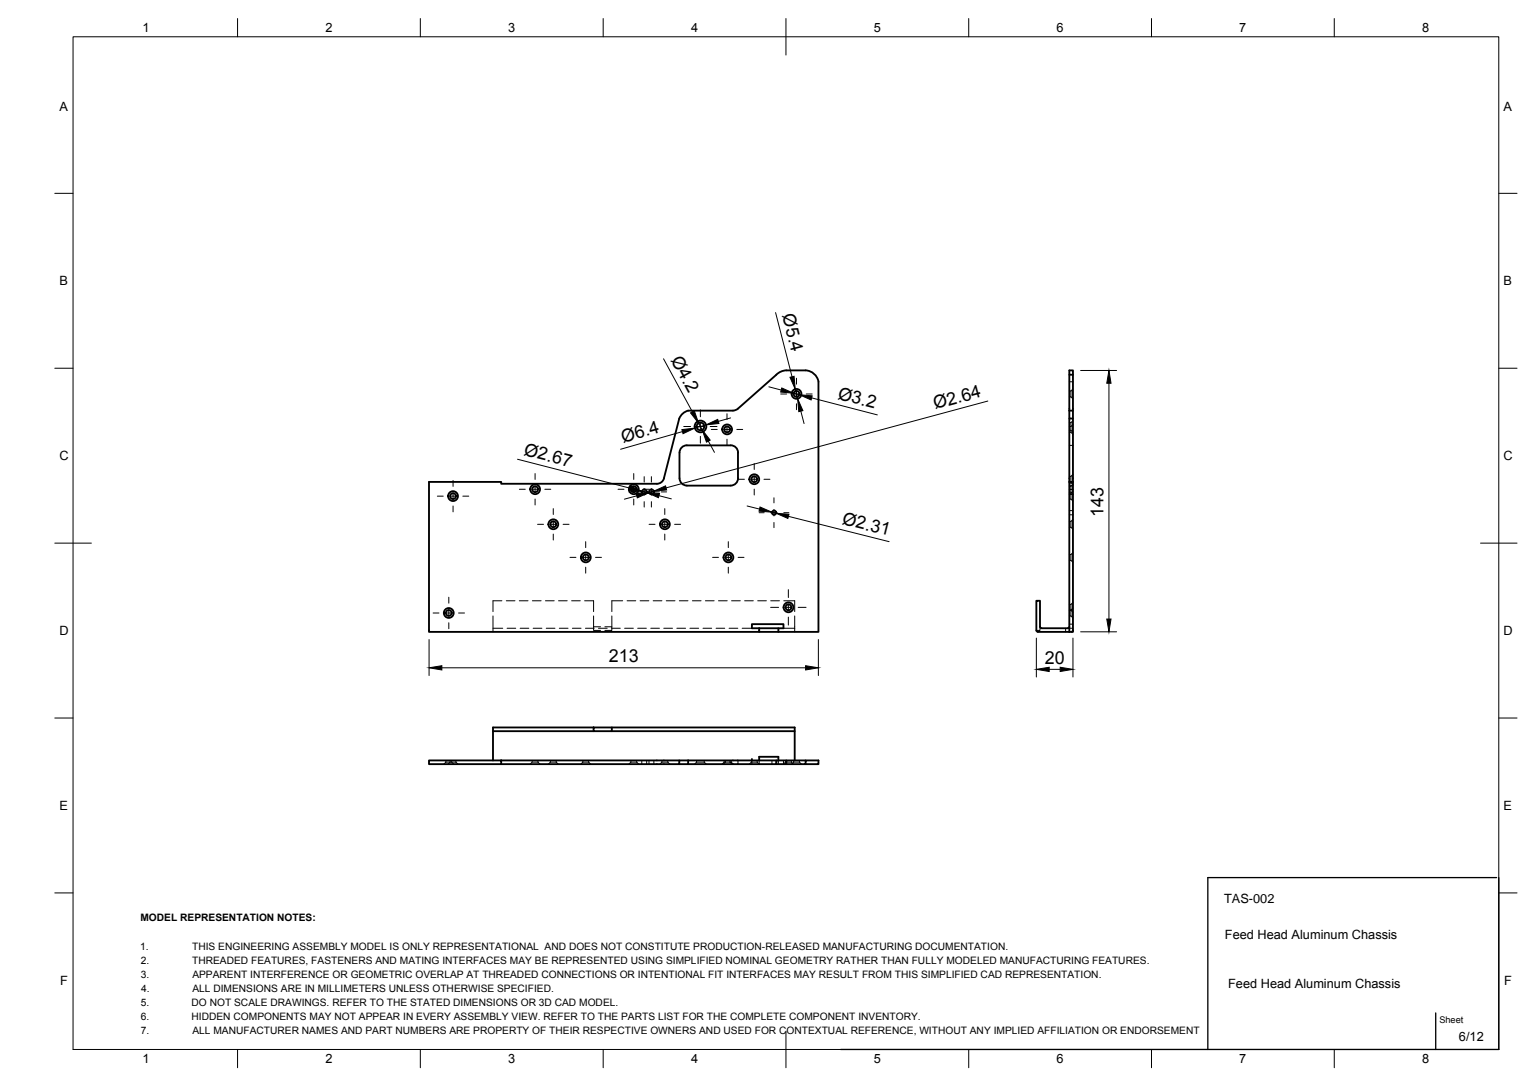
ISO-10303-21;
HEADER;
/* Generated by software containing ST-Developer
 * from STEP Tools, Inc. (www.steptools.com) 
 */

FILE_DESCRIPTION(
/* description */ ('STEP AP214'),
/* implementation_level */ '2;1');

FILE_NAME(
/* name */ 'Feed Head Aluminum Chassis.step',
/* time_stamp */ '2026-11-04T19:38:14-08:00',
/* author */ (''),
/* organization */ (''),
/* preprocessor_version */ 'ST-DEVELOPER v20.2',
/* originating_system */ 'Autodesk Translation Framework v15.17.0.0',
/* authorisation */ '');

FILE_SCHEMA (('AUTOMOTIVE_DESIGN { 1 0 10303 214 3 1 1 }'));
ENDSEC;

DATA;
#10=MECHANICAL_DESIGN_GEOMETRIC_PRESENTATION_REPRESENTATION('',(#473),#36668);
#171=CONICAL_SURFACE('',#18583,1.6,0.785398163397458);
#172=CONICAL_SURFACE('',#18587,1.6,0.785398163397457);
#173=CONICAL_SURFACE('',#18591,1.6,0.785398163397458);
#174=CONICAL_SURFACE('',#18595,1.6,0.785398163397457);
#175=CONICAL_SURFACE('',#18599,1.6,0.785398163397457);
#176=CONICAL_SURFACE('',#18603,1.6,0.785398163397457);
#177=CONICAL_SURFACE('',#18607,1.6,0.785398163397457);
#178=CONICAL_SURFACE('',#18611,1.6,0.785398163397457);
#179=CONICAL_SURFACE('',#18615,1.6,0.785398163397457);
#180=CONICAL_SURFACE('',#18619,2.1,0.785398163397457);
#181=CONICAL_SURFACE('',#18623,1.6,0.785398163397458);
#182=CONICAL_SURFACE('',#18627,1.6,0.785398163397458);
#183=CONICAL_SURFACE('',#18631,1.6,0.785398163397457);
#453=SHAPE_REPRESENTATION_RELATIONSHIP('SRR','None',#36709,#463);
#463=ADVANCED_BREP_SHAPE_REPRESENTATION('',(#483),#36661);
#473=STYLED_ITEM('',(#36768),#483);
#483=MANIFOLD_SOLID_BREP('Body1',#17796);
#585=CYLINDRICAL_SURFACE('',#18565,4.);
#586=CYLINDRICAL_SURFACE('',#18568,4.);
#587=CYLINDRICAL_SURFACE('',#18571,4.);
#588=CYLINDRICAL_SURFACE('',#18574,4.);
#589=CYLINDRICAL_SURFACE('',#18577,4.);
#590=CYLINDRICAL_SURFACE('',#18580,4.);
#591=CYLINDRICAL_SURFACE('',#18644,0.800000000000002);
#592=CYLINDRICAL_SURFACE('',#18646,0.800000000000002);
#593=CYLINDRICAL_SURFACE('',#18648,0.799999999999995);
#594=CYLINDRICAL_SURFACE('',#18651,0.799999999999995);
#595=CYLINDRICAL_SURFACE('',#18661,1.6);
#596=CYLINDRICAL_SURFACE('',#18663,1.15469920262284);
#597=CYLINDRICAL_SURFACE('',#18666,1.6);
#598=CYLINDRICAL_SURFACE('',#18668,1.6);
#599=CYLINDRICAL_SURFACE('',#18670,1.6);
#600=CYLINDRICAL_SURFACE('',#18672,1.33321558059984);
#601=CYLINDRICAL_SURFACE('',#18675,1.32106757713908);
#602=CYLINDRICAL_SURFACE('',#18678,2.1);
#603=CYLINDRICAL_SURFACE('',#18680,1.6);
#604=CYLINDRICAL_SURFACE('',#18682,1.6);
#605=CYLINDRICAL_SURFACE('',#18684,1.6);
#606=CYLINDRICAL_SURFACE('',#18686,1.6);
#607=CYLINDRICAL_SURFACE('',#18688,1.6);
#608=CYLINDRICAL_SURFACE('',#18690,1.6);
#609=CYLINDRICAL_SURFACE('',#18692,1.6);
#610=CYLINDRICAL_SURFACE('',#18694,1.6);
#611=CYLINDRICAL_SURFACE('',#18700,7.25609345692882);
#612=CYLINDRICAL_SURFACE('',#18705,8.3116573007006);
#613=CYLINDRICAL_SURFACE('',#18709,7.62932104676364);
#891=FACE_BOUND('',#2999,.T.);
#892=FACE_BOUND('',#3000,.T.);
#893=FACE_BOUND('',#3001,.T.);
#894=FACE_BOUND('',#3002,.T.);
#895=FACE_BOUND('',#3003,.T.);
#896=FACE_BOUND('',#3004,.T.);
#897=FACE_BOUND('',#3005,.T.);
#898=FACE_BOUND('',#3006,.T.);
#899=FACE_BOUND('',#3007,.T.);
#900=FACE_BOUND('',#3008,.T.);
#901=FACE_BOUND('',#3009,.T.);
#902=FACE_BOUND('',#3010,.T.);
#903=FACE_BOUND('',#3011,.T.);
#904=FACE_BOUND('',#3012,.T.);
#905=FACE_BOUND('',#3013,.T.);
#906=FACE_BOUND('',#3014,.T.);
#907=FACE_BOUND('',#3015,.T.);
#908=FACE_BOUND('',#3017,.T.);
#909=FACE_BOUND('',#3018,.T.);
#910=FACE_BOUND('',#3019,.T.);
#911=FACE_BOUND('',#3020,.T.);
#912=FACE_BOUND('',#3021,.T.);
#913=FACE_BOUND('',#3022,.T.);
#914=FACE_BOUND('',#3023,.T.);
#915=FACE_BOUND('',#3024,.T.);
#916=FACE_BOUND('',#3025,.T.);
#917=FACE_BOUND('',#3026,.T.);
#918=FACE_BOUND('',#3027,.T.);
#919=FACE_BOUND('',#3028,.T.);
#920=FACE_BOUND('',#3029,.T.);
#921=FACE_BOUND('',#3030,.T.);
#922=FACE_BOUND('',#3031,.T.);
#923=FACE_BOUND('',#3032,.T.);
#924=FACE_BOUND('',#3033,.T.);
#1255=CIRCLE('',#18566,4.);
#1256=CIRCLE('',#18567,4.);
#1257=CIRCLE('',#18569,4.);
#1258=CIRCLE('',#18570,4.);
#1259=CIRCLE('',#18572,4.);
#1260=CIRCLE('',#18573,4.);
#1261=CIRCLE('',#18575,4.);
#1262=CIRCLE('',#18576,4.);
#1263=CIRCLE('',#18578,4.);
#1264=CIRCLE('',#18579,4.);
#1265=CIRCLE('',#18581,4.);
#1266=CIRCLE('',#18582,4.);
#1267=CIRCLE('',#18584,1.6);
#1268=CIRCLE('',#18585,1.6);
#1269=CIRCLE('',#18586,2.69999999999999);
#1270=CIRCLE('',#18588,1.6);
#1271=CIRCLE('',#18589,1.6);
#1272=CIRCLE('',#18590,2.69999999999999);
#1273=CIRCLE('',#18592,1.6);
#1274=CIRCLE('',#18593,1.6);
#1275=CIRCLE('',#18594,2.7);
#1276=CIRCLE('',#18596,1.6);
#1277=CIRCLE('',#18597,1.6);
#1278=CIRCLE('',#18598,2.7);
#1279=CIRCLE('',#18600,1.6);
#1280=CIRCLE('',#18601,1.6);
#1281=CIRCLE('',#18602,2.69999999999999);
#1282=CIRCLE('',#18604,1.6);
#1283=CIRCLE('',#18605,1.6);
#1284=CIRCLE('',#18606,2.69999999999995);
#1285=CIRCLE('',#18608,1.6);
#1286=CIRCLE('',#18609,1.6);
#1287=CIRCLE('',#18610,2.7);
#1288=CIRCLE('',#18612,1.6);
#1289=CIRCLE('',#18613,1.6);
#1290=CIRCLE('',#18614,2.69999999999995);
#1291=CIRCLE('',#18616,1.6);
#1292=CIRCLE('',#18617,1.6);
#1293=CIRCLE('',#18618,2.69999999999995);
#1294=CIRCLE('',#18620,2.1);
#1295=CIRCLE('',#18621,2.1);
#1296=CIRCLE('',#18622,3.19999999999996);
#1297=CIRCLE('',#18624,1.6);
#1298=CIRCLE('',#18625,1.6);
#1299=CIRCLE('',#18626,2.7);
#1300=CIRCLE('',#18628,1.6);
#1301=CIRCLE('',#18629,1.6);
#1302=CIRCLE('',#18630,2.7);
#1303=CIRCLE('',#18632,1.6);
#1304=CIRCLE('',#18633,1.6);
#1305=CIRCLE('',#18634,2.69999999999999);
#1306=CIRCLE('',#18637,0.800000000000002);
#1307=CIRCLE('',#18638,0.800000000000002);
#1308=CIRCLE('',#18639,0.800000000000002);
#1309=CIRCLE('',#18645,0.800000000000002);
#1310=CIRCLE('',#18647,0.800000000000002);
#1311=CIRCLE('',#18649,0.800000000000002);
#1312=CIRCLE('',#18650,0.799999999999995);
#1313=CIRCLE('',#18652,0.800000000000002);
#1314=CIRCLE('',#18662,1.6);
#1315=CIRCLE('',#18664,1.15469920262284);
#1316=CIRCLE('',#18665,1.15469920262284);
#1317=CIRCLE('',#18667,1.6);
#1318=CIRCLE('',#18669,1.6);
#1319=CIRCLE('',#18671,1.6);
#1320=CIRCLE('',#18673,1.33321558059984);
#1321=CIRCLE('',#18674,1.33321558059984);
#1322=CIRCLE('',#18676,1.32106757713908);
#1323=CIRCLE('',#18677,1.32106757713908);
#1324=CIRCLE('',#18679,2.1);
#1325=CIRCLE('',#18681,1.6);
#1326=CIRCLE('',#18683,1.6);
#1327=CIRCLE('',#18685,1.6);
#1328=CIRCLE('',#18687,1.6);
#1329=CIRCLE('',#18689,1.6);
#1330=CIRCLE('',#18691,1.6);
#1331=CIRCLE('',#18693,1.6);
#1332=CIRCLE('',#18695,1.6);
#1333=CIRCLE('',#18701,7.25609345692882);
#1334=CIRCLE('',#18702,7.25609345692882);
#1335=CIRCLE('',#18706,8.3116573007006);
#1336=CIRCLE('',#18707,8.3116573007006);
#1337=CIRCLE('',#18710,7.62932104676364);
#1338=CIRCLE('',#18711,7.62932104676364);
#1880=FACE_OUTER_BOUND('',#2926,.T.);
#1881=FACE_OUTER_BOUND('',#2927,.T.);
#1882=FACE_OUTER_BOUND('',#2928,.T.);
#1883=FACE_OUTER_BOUND('',#2929,.T.);
#1884=FACE_OUTER_BOUND('',#2930,.T.);
#1885=FACE_OUTER_BOUND('',#2931,.T.);
#1886=FACE_OUTER_BOUND('',#2932,.T.);
#1887=FACE_OUTER_BOUND('',#2933,.T.);
#1888=FACE_OUTER_BOUND('',#2934,.T.);
#1889=FACE_OUTER_BOUND('',#2935,.T.);
#1890=FACE_OUTER_BOUND('',#2936,.T.);
#1891=FACE_OUTER_BOUND('',#2937,.T.);
#1892=FACE_OUTER_BOUND('',#2938,.T.);
#1893=FACE_OUTER_BOUND('',#2939,.T.);
#1894=FACE_OUTER_BOUND('',#2940,.T.);
#1895=FACE_OUTER_BOUND('',#2941,.T.);
#1896=FACE_OUTER_BOUND('',#2942,.T.);
#1897=FACE_OUTER_BOUND('',#2943,.T.);
#1898=FACE_OUTER_BOUND('',#2944,.T.);
#1899=FACE_OUTER_BOUND('',#2945,.T.);
#1900=FACE_OUTER_BOUND('',#2946,.T.);
#1901=FACE_OUTER_BOUND('',#2947,.T.);
#1902=FACE_OUTER_BOUND('',#2948,.T.);
#1903=FACE_OUTER_BOUND('',#2949,.T.);
#1904=FACE_OUTER_BOUND('',#2950,.T.);
#1905=FACE_OUTER_BOUND('',#2951,.T.);
#1906=FACE_OUTER_BOUND('',#2952,.T.);
#1907=FACE_OUTER_BOUND('',#2953,.T.);
#1908=FACE_OUTER_BOUND('',#2954,.T.);
#1909=FACE_OUTER_BOUND('',#2955,.T.);
#1910=FACE_OUTER_BOUND('',#2956,.T.);
#1911=FACE_OUTER_BOUND('',#2957,.T.);
#1912=FACE_OUTER_BOUND('',#2958,.T.);
#1913=FACE_OUTER_BOUND('',#2959,.T.);
#1914=FACE_OUTER_BOUND('',#2960,.T.);
#1915=FACE_OUTER_BOUND('',#2961,.T.);
#1916=FACE_OUTER_BOUND('',#2962,.T.);
#1917=FACE_OUTER_BOUND('',#2963,.T.);
#1918=FACE_OUTER_BOUND('',#2964,.T.);
#1919=FACE_OUTER_BOUND('',#2965,.T.);
#1920=FACE_OUTER_BOUND('',#2966,.T.);
#1921=FACE_OUTER_BOUND('',#2967,.T.);
#1922=FACE_OUTER_BOUND('',#2968,.T.);
#1923=FACE_OUTER_BOUND('',#2969,.T.);
#1924=FACE_OUTER_BOUND('',#2970,.T.);
#1925=FACE_OUTER_BOUND('',#2971,.T.);
#1926=FACE_OUTER_BOUND('',#2972,.T.);
#1927=FACE_OUTER_BOUND('',#2973,.T.);
#1928=FACE_OUTER_BOUND('',#2974,.T.);
#1929=FACE_OUTER_BOUND('',#2975,.T.);
#1930=FACE_OUTER_BOUND('',#2976,.T.);
#1931=FACE_OUTER_BOUND('',#2977,.T.);
#1932=FACE_OUTER_BOUND('',#2978,.T.);
#1933=FACE_OUTER_BOUND('',#2979,.T.);
#1934=FACE_OUTER_BOUND('',#2980,.T.);
#1935=FACE_OUTER_BOUND('',#2981,.T.);
#1936=FACE_OUTER_BOUND('',#2982,.T.);
#1937=FACE_OUTER_BOUND('',#2983,.T.);
#1938=FACE_OUTER_BOUND('',#2984,.T.);
#1939=FACE_OUTER_BOUND('',#2985,.T.);
#1940=FACE_OUTER_BOUND('',#2986,.T.);
#1941=FACE_OUTER_BOUND('',#2987,.T.);
#1942=FACE_OUTER_BOUND('',#2988,.T.);
#1943=FACE_OUTER_BOUND('',#2989,.T.);
#1944=FACE_OUTER_BOUND('',#2990,.T.);
#1945=FACE_OUTER_BOUND('',#2991,.T.);
#1946=FACE_OUTER_BOUND('',#2992,.T.);
#1947=FACE_OUTER_BOUND('',#2993,.T.);
#1948=FACE_OUTER_BOUND('',#2994,.T.);
#1949=FACE_OUTER_BOUND('',#2995,.T.);
#1950=FACE_OUTER_BOUND('',#2996,.T.);
#1951=FACE_OUTER_BOUND('',#2997,.T.);
#1952=FACE_OUTER_BOUND('',#2998,.T.);
#1953=FACE_OUTER_BOUND('',#3016,.T.);
#1954=FACE_OUTER_BOUND('',#3034,.T.);
#1955=FACE_OUTER_BOUND('',#3035,.T.);
#1956=FACE_OUTER_BOUND('',#3036,.T.);
#2926=EDGE_LOOP('',(#13188,#13189,#13190,#13191));
#2927=EDGE_LOOP('',(#13192,#13193,#13194,#13195));
#2928=EDGE_LOOP('',(#13196,#13197,#13198,#13199));
#2929=EDGE_LOOP('',(#13200,#13201,#13202,#13203));
#2930=EDGE_LOOP('',(#13204,#13205,#13206,#13207));
#2931=EDGE_LOOP('',(#13208,#13209,#13210,#13211));
#2932=EDGE_LOOP('',(#13212,#13213,#13214,#13215,#13216));
#2933=EDGE_LOOP('',(#13217,#13218,#13219,#13220,#13221));
#2934=EDGE_LOOP('',(#13222,#13223,#13224,#13225,#13226));
#2935=EDGE_LOOP('',(#13227,#13228,#13229,#13230,#13231));
#2936=EDGE_LOOP('',(#13232,#13233,#13234,#13235,#13236));
#2937=EDGE_LOOP('',(#13237,#13238,#13239,#13240,#13241));
#2938=EDGE_LOOP('',(#13242,#13243,#13244,#13245,#13246));
#2939=EDGE_LOOP('',(#13247,#13248,#13249,#13250,#13251));
#2940=EDGE_LOOP('',(#13252,#13253,#13254,#13255,#13256));
#2941=EDGE_LOOP('',(#13257,#13258,#13259,#13260,#13261));
#2942=EDGE_LOOP('',(#13262,#13263,#13264,#13265,#13266));
#2943=EDGE_LOOP('',(#13267,#13268,#13269,#13270,#13271));
#2944=EDGE_LOOP('',(#13272,#13273,#13274,#13275,#13276));
#2945=EDGE_LOOP('',(#13277,#13278,#13279,#13280));
#2946=EDGE_LOOP('',(#13281,#13282,#13283,#13284,#13285,#13286,#13287,#13288,
#13289));
#2947=EDGE_LOOP('',(#13290,#13291,#13292,#13293));
#2948=EDGE_LOOP('',(#13294,#13295,#13296,#13297,#13298));
#2949=EDGE_LOOP('',(#13299,#13300,#13301,#13302));
#2950=EDGE_LOOP('',(#13303,#13304,#13305,#13306,#13307));
#2951=EDGE_LOOP('',(#13308,#13309,#13310,#13311));
#2952=EDGE_LOOP('',(#13312,#13313,#13314,#13315,#13316,#13317));
#2953=EDGE_LOOP('',(#13318,#13319,#13320,#13321));
#2954=EDGE_LOOP('',(#13322,#13323,#13324,#13325,#13326,#13327));
#2955=EDGE_LOOP('',(#13328,#13329,#13330,#13331,#13332,#13333,#13334,#13335));
#2956=EDGE_LOOP('',(#13336,#13337,#13338,#13339));
#2957=EDGE_LOOP('',(#13340,#13341,#13342,#13343));
#2958=EDGE_LOOP('',(#13344,#13345,#13346,#13347));
#2959=EDGE_LOOP('',(#13348,#13349,#13350,#13351));
#2960=EDGE_LOOP('',(#13352,#13353,#13354,#13355));
#2961=EDGE_LOOP('',(#13356,#13357,#13358,#13359));
#2962=EDGE_LOOP('',(#13360,#13361,#13362,#13363));
#2963=EDGE_LOOP('',(#13364,#13365,#13366,#13367,#13368));
#2964=EDGE_LOOP('',(#13369,#13370,#13371,#13372));
#2965=EDGE_LOOP('',(#13373,#13374,#13375,#13376,#13377));
#2966=EDGE_LOOP('',(#13378,#13379,#13380,#13381,#13382));
#2967=EDGE_LOOP('',(#13383,#13384,#13385,#13386,#13387));
#2968=EDGE_LOOP('',(#13388,#13389,#13390,#13391));
#2969=EDGE_LOOP('',(#13392,#13393,#13394,#13395));
#2970=EDGE_LOOP('',(#13396,#13397,#13398,#13399,#13400));
#2971=EDGE_LOOP('',(#13401,#13402,#13403,#13404,#13405));
#2972=EDGE_LOOP('',(#13406,#13407,#13408,#13409,#13410));
#2973=EDGE_LOOP('',(#13411,#13412,#13413,#13414,#13415));
#2974=EDGE_LOOP('',(#13416,#13417,#13418,#13419,#13420));
#2975=EDGE_LOOP('',(#13421,#13422,#13423,#13424,#13425));
#2976=EDGE_LOOP('',(#13426,#13427,#13428,#13429,#13430));
#2977=EDGE_LOOP('',(#13431,#13432,#13433,#13434,#13435));
#2978=EDGE_LOOP('',(#13436,#13437,#13438,#13439,#13440));
#2979=EDGE_LOOP('',(#13441,#13442,#13443,#13444));
#2980=EDGE_LOOP('',(#13445,#13446,#13447,#13448));
#2981=EDGE_LOOP('',(#13449,#13450,#13451,#13452));
#2982=EDGE_LOOP('',(#13453,#13454,#13455,#13456));
#2983=EDGE_LOOP('',(#13457,#13458,#13459,#13460));
#2984=EDGE_LOOP('',(#13461,#13462,#13463,#13464));
#2985=EDGE_LOOP('',(#13465,#13466,#13467,#13468));
#2986=EDGE_LOOP('',(#13469,#13470,#13471,#13472));
#2987=EDGE_LOOP('',(#13473,#13474,#13475,#13476));
#2988=EDGE_LOOP('',(#13477,#13478,#13479,#13480));
#2989=EDGE_LOOP('',(#13481,#13482,#13483,#13484));
#2990=EDGE_LOOP('',(#13485,#13486,#13487,#13488,#13489,#13490,#13491,#13492,
#13493,#13494,#13495,#13496));
#2991=EDGE_LOOP('',(#13497,#13498,#13499,#13500));
#2992=EDGE_LOOP('',(#13501,#13502,#13503,#13504,#13505,#13506,#13507,#13508,
#13509,#13510,#13511,#13512));
#2993=EDGE_LOOP('',(#13513,#13514,#13515,#13516));
#2994=EDGE_LOOP('',(#13517,#13518,#13519,#13520));
#2995=EDGE_LOOP('',(#13521,#13522,#13523,#13524,#13525));
#2996=EDGE_LOOP('',(#13526,#13527,#13528,#13529,#13530));
#2997=EDGE_LOOP('',(#13531,#13532,#13533,#13534,#13535));
#2998=EDGE_LOOP('',(#13536,#13537,#13538,#13539,#13540,#13541,#13542,#13543,
#13544,#13545,#13546,#13547,#13548,#13549,#13550,#13551,#13552,#13553,#13554,
#13555,#13556,#13557,#13558));
#2999=EDGE_LOOP('',(#13559));
#3000=EDGE_LOOP('',(#13560,#13561,#13562,#13563,#13564,#13565,#13566,#13567));
#3001=EDGE_LOOP('',(#13568));
#3002=EDGE_LOOP('',(#13569));
#3003=EDGE_LOOP('',(#13570));
#3004=EDGE_LOOP('',(#13571));
#3005=EDGE_LOOP('',(#13572));
#3006=EDGE_LOOP('',(#13573));
#3007=EDGE_LOOP('',(#13574));
#3008=EDGE_LOOP('',(#13575));
#3009=EDGE_LOOP('',(#13576));
#3010=EDGE_LOOP('',(#13577));
#3011=EDGE_LOOP('',(#13578));
#3012=EDGE_LOOP('',(#13579));
#3013=EDGE_LOOP('',(#13580));
#3014=EDGE_LOOP('',(#13581));
#3015=EDGE_LOOP('',(#13582));
#3016=EDGE_LOOP('',(#13583,#13584,#13585,#13586,#13587,#13588,#13589,#13590,
#13591,#13592,#13593,#13594,#13595,#13596,#13597,#13598,#13599,#13600,#13601,
#13602,#13603,#13604,#13605));
#3017=EDGE_LOOP('',(#13606,#13607,#13608,#13609,#13610,#13611,#13612,#13613));
#3018=EDGE_LOOP('',(#13614));
#3019=EDGE_LOOP('',(#13615));
#3020=EDGE_LOOP('',(#13616));
#3021=EDGE_LOOP('',(#13617));
#3022=EDGE_LOOP('',(#13618));
#3023=EDGE_LOOP('',(#13619));
#3024=EDGE_LOOP('',(#13620));
#3025=EDGE_LOOP('',(#13621));
#3026=EDGE_LOOP('',(#13622));
#3027=EDGE_LOOP('',(#13623));
#3028=EDGE_LOOP('',(#13624));
#3029=EDGE_LOOP('',(#13625));
#3030=EDGE_LOOP('',(#13626));
#3031=EDGE_LOOP('',(#13627));
#3032=EDGE_LOOP('',(#13628));
#3033=EDGE_LOOP('',(#13629));
#3034=EDGE_LOOP('',(#13630,#13631,#13632,#13633));
#3035=EDGE_LOOP('',(#13634,#13635,#13636,#13637));
#3036=EDGE_LOOP('',(#13638,#13639,#13640,#13641));
#4229=LINE('',#26847,#5939);
#4230=LINE('',#26850,#5940);
#4231=LINE('',#26856,#5941);
#4232=LINE('',#26859,#5942);
#4233=LINE('',#26865,#5943);
#4234=LINE('',#26868,#5944);
#4235=LINE('',#26874,#5945);
#4236=LINE('',#26877,#5946);
#4237=LINE('',#26883,#5947);
#4238=LINE('',#26886,#5948);
#4239=LINE('',#26892,#5949);
#4240=LINE('',#26895,#5950);
#4241=LINE('',#26902,#5951);
#4242=LINE('',#26910,#5952);
#4243=LINE('',#26918,#5953);
#4244=LINE('',#26926,#5954);
#4245=LINE('',#26934,#5955);
#4246=LINE('',#26942,#5956);
#4247=LINE('',#26950,#5957);
#4248=LINE('',#26958,#5958);
#4249=LINE('',#26966,#5959);
#4250=LINE('',#26974,#5960);
#4251=LINE('',#26982,#5961);
#4252=LINE('',#26990,#5962);
#4253=LINE('',#26998,#5963);
#4254=LINE('',#27003,#5964);
#4255=LINE('',#27005,#5965);
#4256=LINE('',#27007,#5966);
#4257=LINE('',#27008,#5967);
#4258=LINE('',#27014,#5968);
#4259=LINE('',#27016,#5969);
#4260=LINE('',#27020,#5970);
#4261=LINE('',#27024,#5971);
#4262=LINE('',#27026,#5972);
#4263=LINE('',#27027,#5973);
#4264=LINE('',#27031,#5974);
#4265=LINE('',#27033,#5975);
#4266=LINE('',#27035,#5976);
#4267=LINE('',#27036,#5977);
#4268=LINE('',#27040,#5978);
#4269=LINE('',#27041,#5979);
#4270=LINE('',#27043,#5980);
#4271=LINE('',#27044,#5981);
#4272=LINE('',#27047,#5982);
#4273=LINE('',#27048,#5983);
#4274=LINE('',#27051,#5984);
#4275=LINE('',#27053,#5985);
#4276=LINE('',#27054,#5986);
#4277=LINE('',#27057,#5987);
#4278=LINE('',#27059,#5988);
#4279=LINE('',#27062,#5989);
#4280=LINE('',#27064,#5990);
#4281=LINE('',#27067,#5991);
#4282=LINE('',#27073,#5992);
#4283=LINE('',#27076,#5993);
#4284=LINE('',#27078,#5994);
#4285=LINE('',#27080,#5995);
#4286=LINE('',#27083,#5996);
#4287=LINE('',#27086,#5997);
#4288=LINE('',#27088,#5998);
#4289=LINE('',#27090,#5999);
#4290=LINE('',#27091,#6000);
#4291=LINE('',#27093,#6001);
#4292=LINE('',#27094,#6002);
#4293=LINE('',#27096,#6003);
#4294=LINE('',#27098,#6004);
#4295=LINE('',#27101,#6005);
#4296=LINE('',#27102,#6006);
#4297=LINE('',#27104,#6007);
#4298=LINE('',#27105,#6008);
#4299=LINE('',#27107,#6009);
#4300=LINE('',#27108,#6010);
#4301=LINE('',#27110,#6011);
#4302=LINE('',#27111,#6012);
#4303=LINE('',#27114,#6013);
#4304=LINE('',#27120,#6014);
#4305=LINE('',#27124,#6015);
#4306=LINE('',#27128,#6016);
#4307=LINE('',#27132,#6017);
#4308=LINE('',#27138,#6018);
#4309=LINE('',#27144,#6019);
#4310=LINE('',#27148,#6020);
#4311=LINE('',#27152,#6021);
#4312=LINE('',#27156,#6022);
#4313=LINE('',#27160,#6023);
#4314=LINE('',#27164,#6024);
#4315=LINE('',#27168,#6025);
#4316=LINE('',#27172,#6026);
#4317=LINE('',#27176,#6027);
#4318=LINE('',#27180,#6028);
#4319=LINE('',#27185,#6029);
#4320=LINE('',#27187,#6030);
#4321=LINE('',#27189,#6031);
#4322=LINE('',#27190,#6032);
#4323=LINE('',#27193,#6033);
#4324=LINE('',#27195,#6034);
#4325=LINE('',#27196,#6035);
#4326=LINE('',#27198,#6036);
#4327=LINE('',#27199,#6037);
#4328=LINE('',#27202,#6038);
#4329=LINE('',#27204,#6039);
#4330=LINE('',#27205,#6040);
#4331=LINE('',#27211,#6041);
#4332=LINE('',#27213,#6042);
#4333=LINE('',#27214,#6043);
#4334=LINE('',#27217,#6044);
#4335=LINE('',#27219,#6045);
#4336=LINE('',#27220,#6046);
#4337=LINE('',#27226,#6047);
#4338=LINE('',#27229,#6048);
#4339=LINE('',#27231,#6049);
#4340=LINE('',#27232,#6050);
#4341=LINE('',#27238,#6051);
#4342=LINE('',#27241,#6052);
#4343=LINE('',#27243,#6053);
#4344=LINE('',#27244,#6054);
#4345=LINE('',#27246,#6055);
#4346=LINE('',#27248,#6056);
#4347=LINE('',#27249,#6057);
#4348=LINE('',#27250,#6058);
#4349=LINE('',#27252,#6059);
#4350=LINE('',#27253,#6060);
#4351=LINE('',#27256,#6061);
#4352=LINE('',#27257,#6062);
#4353=LINE('',#27260,#6063);
#4354=LINE('',#27262,#6064);
#4355=LINE('',#27264,#6065);
#4356=LINE('',#27265,#6066);
#4357=LINE('',#27267,#6067);
#4358=LINE('',#27268,#6068);
#4359=LINE('',#27271,#6069);
#4360=LINE('',#27273,#6070);
#4361=LINE('',#27274,#6071);
#4362=LINE('',#27277,#6072);
#4363=LINE('',#27279,#6073);
#4364=LINE('',#27280,#6074);
#4365=LINE('',#27282,#6075);
#4366=LINE('',#27283,#6076);
#4367=LINE('',#27285,#6077);
#4368=LINE('',#27287,#6078);
#4369=LINE('',#27288,#6079);
#4370=LINE('',#27292,#6080);
#4371=LINE('',#27294,#6081);
#5939=VECTOR('',#21385,1000.);
#5940=VECTOR('',#21388,1000.);
#5941=VECTOR('',#21393,1000.);
#5942=VECTOR('',#21396,1000.);
#5943=VECTOR('',#21401,1000.);
#5944=VECTOR('',#21404,1000.);
#5945=VECTOR('',#21409,1000.);
#5946=VECTOR('',#21412,1000.);
#5947=VECTOR('',#21417,1000.);
#5948=VECTOR('',#21420,1000.);
#5949=VECTOR('',#21425,1000.);
#5950=VECTOR('',#21428,1000.);
#5951=VECTOR('',#21435,1.6);
#5952=VECTOR('',#21444,1.6);
#5953=VECTOR('',#21453,1.6);
#5954=VECTOR('',#21462,1.6);
#5955=VECTOR('',#21471,1.6);
#5956=VECTOR('',#21480,1.6);
#5957=VECTOR('',#21489,1.6);
#5958=VECTOR('',#21498,1.6);
#5959=VECTOR('',#21507,1.6);
#5960=VECTOR('',#21516,2.1);
#5961=VECTOR('',#21525,1.6);
#5962=VECTOR('',#21534,1.6);
#5963=VECTOR('',#21543,1.6);
#5964=VECTOR('',#21548,1000.);
#5965=VECTOR('',#21549,1000.);
#5966=VECTOR('',#21550,1000.);
#5967=VECTOR('',#21551,1000.);
#5968=VECTOR('',#21556,1000.);
#5969=VECTOR('',#21557,1000.);
#5970=VECTOR('',#21560,1000.);
#5971=VECTOR('',#21563,1000.);
#5972=VECTOR('',#21564,1000.);
#5973=VECTOR('',#21565,1000.);
#5974=VECTOR('',#21568,1000.);
#5975=VECTOR('',#21569,1000.);
#5976=VECTOR('',#21570,1000.);
#5977=VECTOR('',#21571,1000.);
#5978=VECTOR('',#21574,1000.);
#5979=VECTOR('',#21575,1000.);
#5980=VECTOR('',#21576,1000.);
#5981=VECTOR('',#21577,1000.);
#5982=VECTOR('',#21580,1000.);
#5983=VECTOR('',#21581,1000.);
#5984=VECTOR('',#21584,1000.);
#5985=VECTOR('',#21585,1000.);
#5986=VECTOR('',#21586,1000.);
#5987=VECTOR('',#21589,1000.);
#5988=VECTOR('',#21590,1000.);
#5989=VECTOR('',#21595,1000.);
#5990=VECTOR('',#21596,1000.);
#5991=VECTOR('',#21599,1000.);
#5992=VECTOR('',#21604,1000.);
#5993=VECTOR('',#21607,1000.);
#5994=VECTOR('',#21610,1000.);
#5995=VECTOR('',#21611,1000.);
#5996=VECTOR('',#21614,1000.);
#5997=VECTOR('',#21617,1000.);
#5998=VECTOR('',#21618,1000.);
#5999=VECTOR('',#21619,1000.);
#6000=VECTOR('',#21620,1000.);
#6001=VECTOR('',#21621,1000.);
#6002=VECTOR('',#21622,1000.);
#6003=VECTOR('',#21625,1000.);
#6004=VECTOR('',#21628,1000.);
#6005=VECTOR('',#21633,1000.);
#6006=VECTOR('',#21634,1000.);
#6007=VECTOR('',#21637,1000.);
#6008=VECTOR('',#21638,1000.);
#6009=VECTOR('',#21641,1000.);
#6010=VECTOR('',#21642,1000.);
#6011=VECTOR('',#21645,1000.);
#6012=VECTOR('',#21646,1000.);
#6013=VECTOR('',#21649,1.6);
#6014=VECTOR('',#21656,1.15469920262284);
#6015=VECTOR('',#21661,1.6);
#6016=VECTOR('',#21666,1.6);
#6017=VECTOR('',#21671,1.6);
#6018=VECTOR('',#21678,1.33321558059984);
#6019=VECTOR('',#21685,1.32106757713908);
#6020=VECTOR('',#21690,2.1);
#6021=VECTOR('',#21695,1.6);
#6022=VECTOR('',#21700,1.6);
#6023=VECTOR('',#21705,1.6);
#6024=VECTOR('',#21710,1.6);
#6025=VECTOR('',#21715,1.6);
#6026=VECTOR('',#21720,1.6);
#6027=VECTOR('',#21725,1.6);
#6028=VECTOR('',#21730,1.6);
#6029=VECTOR('',#21735,1000.);
#6030=VECTOR('',#21736,1000.);
#6031=VECTOR('',#21737,1000.);
#6032=VECTOR('',#21738,1000.);
#6033=VECTOR('',#21741,1000.);
#6034=VECTOR('',#21742,1000.);
#6035=VECTOR('',#21743,1000.);
#6036=VECTOR('',#21746,1000.);
#6037=VECTOR('',#21747,1000.);
#6038=VECTOR('',#21750,1000.);
#6039=VECTOR('',#21751,1000.);
#6040=VECTOR('',#21752,1000.);
#6041=VECTOR('',#21759,1000.);
#6042=VECTOR('',#21762,1000.);
#6043=VECTOR('',#21763,1000.);
#6044=VECTOR('',#21766,1000.);
#6045=VECTOR('',#21767,1000.);
#6046=VECTOR('',#21768,1000.);
#6047=VECTOR('',#21775,1000.);
#6048=VECTOR('',#21778,1000.);
#6049=VECTOR('',#21779,1000.);
#6050=VECTOR('',#21780,1000.);
#6051=VECTOR('',#21787,1000.);
#6052=VECTOR('',#21790,1000.);
#6053=VECTOR('',#21791,1000.);
#6054=VECTOR('',#21792,1000.);
#6055=VECTOR('',#21795,1000.);
#6056=VECTOR('',#21796,1000.);
#6057=VECTOR('',#21797,1000.);
#6058=VECTOR('',#21798,1000.);
#6059=VECTOR('',#21799,1000.);
#6060=VECTOR('',#21800,1000.);
#6061=VECTOR('',#21803,1000.);
#6062=VECTOR('',#21804,1000.);
#6063=VECTOR('',#21807,1000.);
#6064=VECTOR('',#21808,1000.);
#6065=VECTOR('',#21809,1000.);
#6066=VECTOR('',#21810,1000.);
#6067=VECTOR('',#21811,1000.);
#6068=VECTOR('',#21812,1000.);
#6069=VECTOR('',#21815,1000.);
#6070=VECTOR('',#21816,1000.);
#6071=VECTOR('',#21817,1000.);
#6072=VECTOR('',#21820,1000.);
#6073=VECTOR('',#21821,1000.);
#6074=VECTOR('',#21822,1000.);
#6075=VECTOR('',#21825,1000.);
#6076=VECTOR('',#21826,1000.);
#6077=VECTOR('',#21829,1000.);
#6078=VECTOR('',#21832,1000.);
#6079=VECTOR('',#21833,1000.);
#6080=VECTOR('',#21840,1000.);
#6081=VECTOR('',#21843,1000.);
#7633=VERTEX_POINT('',#26843);
#7634=VERTEX_POINT('',#26844);
#7635=VERTEX_POINT('',#26846);
#7636=VERTEX_POINT('',#26848);
#7637=VERTEX_POINT('',#26852);
#7638=VERTEX_POINT('',#26853);
#7639=VERTEX_POINT('',#26855);
#7640=VERTEX_POINT('',#26857);
#7641=VERTEX_POINT('',#26861);
#7642=VERTEX_POINT('',#26862);
#7643=VERTEX_POINT('',#26864);
#7644=VERTEX_POINT('',#26866);
#7645=VERTEX_POINT('',#26870);
#7646=VERTEX_POINT('',#26871);
#7647=VERTEX_POINT('',#26873);
#7648=VERTEX_POINT('',#26875);
#7649=VERTEX_POINT('',#26879);
#7650=VERTEX_POINT('',#26880);
#7651=VERTEX_POINT('',#26882);
#7652=VERTEX_POINT('',#26884);
#7653=VERTEX_POINT('',#26888);
#7654=VERTEX_POINT('',#26889);
#7655=VERTEX_POINT('',#26891);
#7656=VERTEX_POINT('',#26893);
#7657=VERTEX_POINT('',#26897);
#7658=VERTEX_POINT('',#26898);
#7659=VERTEX_POINT('',#26901);
#7660=VERTEX_POINT('',#26905);
#7661=VERTEX_POINT('',#26906);
#7662=VERTEX_POINT('',#26909);
#7663=VERTEX_POINT('',#26913);
#7664=VERTEX_POINT('',#26914);
#7665=VERTEX_POINT('',#26917);
#7666=VERTEX_POINT('',#26921);
#7667=VERTEX_POINT('',#26922);
#7668=VERTEX_POINT('',#26925);
#7669=VERTEX_POINT('',#26929);
#7670=VERTEX_POINT('',#26930);
#7671=VERTEX_POINT('',#26933);
#7672=VERTEX_POINT('',#26937);
#7673=VERTEX_POINT('',#26938);
#7674=VERTEX_POINT('',#26941);
#7675=VERTEX_POINT('',#26945);
#7676=VERTEX_POINT('',#26946);
#7677=VERTEX_POINT('',#26949);
#7678=VERTEX_POINT('',#26953);
#7679=VERTEX_POINT('',#26954);
#7680=VERTEX_POINT('',#26957);
#7681=VERTEX_POINT('',#26961);
#7682=VERTEX_POINT('',#26962);
#7683=VERTEX_POINT('',#26965);
#7684=VERTEX_POINT('',#26969);
#7685=VERTEX_POINT('',#26970);
#7686=VERTEX_POINT('',#26973);
#7687=VERTEX_POINT('',#26977);
#7688=VERTEX_POINT('',#26978);
#7689=VERTEX_POINT('',#26981);
#7690=VERTEX_POINT('',#26985);
#7691=VERTEX_POINT('',#26986);
#7692=VERTEX_POINT('',#26989);
#7693=VERTEX_POINT('',#26993);
#7694=VERTEX_POINT('',#26994);
#7695=VERTEX_POINT('',#26997);
#7696=VERTEX_POINT('',#27001);
#7697=VERTEX_POINT('',#27002);
#7698=VERTEX_POINT('',#27004);
#7699=VERTEX_POINT('',#27006);
#7700=VERTEX_POINT('',#27010);
#7701=VERTEX_POINT('',#27011);
#7702=VERTEX_POINT('',#27013);
#7703=VERTEX_POINT('',#27015);
#7704=VERTEX_POINT('',#27017);
#7705=VERTEX_POINT('',#27019);
#7706=VERTEX_POINT('',#27021);
#7707=VERTEX_POINT('',#27023);
#7708=VERTEX_POINT('',#27025);
#7709=VERTEX_POINT('',#27029);
#7710=VERTEX_POINT('',#27030);
#7711=VERTEX_POINT('',#27032);
#7712=VERTEX_POINT('',#27034);
#7713=VERTEX_POINT('',#27038);
#7714=VERTEX_POINT('',#27039);
#7715=VERTEX_POINT('',#27042);
#7716=VERTEX_POINT('',#27046);
#7717=VERTEX_POINT('',#27050);
#7718=VERTEX_POINT('',#27052);
#7719=VERTEX_POINT('',#27056);
#7720=VERTEX_POINT('',#27058);
#7721=VERTEX_POINT('',#27063);
#7722=VERTEX_POINT('',#27065);
#7723=VERTEX_POINT('',#27069);
#7724=VERTEX_POINT('',#27070);
#7725=VERTEX_POINT('',#27072);
#7726=VERTEX_POINT('',#27074);
#7727=VERTEX_POINT('',#27079);
#7728=VERTEX_POINT('',#27081);
#7729=VERTEX_POINT('',#27085);
#7730=VERTEX_POINT('',#27087);
#7731=VERTEX_POINT('',#27089);
#7732=VERTEX_POINT('',#27092);
#7733=VERTEX_POINT('',#27113);
#7734=VERTEX_POINT('',#27117);
#7735=VERTEX_POINT('',#27119);
#7736=VERTEX_POINT('',#27123);
#7737=VERTEX_POINT('',#27127);
#7738=VERTEX_POINT('',#27131);
#7739=VERTEX_POINT('',#27135);
#7740=VERTEX_POINT('',#27137);
#7741=VERTEX_POINT('',#27141);
#7742=VERTEX_POINT('',#27143);
#7743=VERTEX_POINT('',#27147);
#7744=VERTEX_POINT('',#27151);
#7745=VERTEX_POINT('',#27155);
#7746=VERTEX_POINT('',#27159);
#7747=VERTEX_POINT('',#27163);
#7748=VERTEX_POINT('',#27167);
#7749=VERTEX_POINT('',#27171);
#7750=VERTEX_POINT('',#27175);
#7751=VERTEX_POINT('',#27179);
#7752=VERTEX_POINT('',#27183);
#7753=VERTEX_POINT('',#27184);
#7754=VERTEX_POINT('',#27186);
#7755=VERTEX_POINT('',#27188);
#7756=VERTEX_POINT('',#27192);
#7757=VERTEX_POINT('',#27194);
#7758=VERTEX_POINT('',#27201);
#7759=VERTEX_POINT('',#27203);
#7760=VERTEX_POINT('',#27207);
#7761=VERTEX_POINT('',#27209);
#7762=VERTEX_POINT('',#27216);
#7763=VERTEX_POINT('',#27218);
#7764=VERTEX_POINT('',#27222);
#7765=VERTEX_POINT('',#27224);
#7766=VERTEX_POINT('',#27228);
#7767=VERTEX_POINT('',#27230);
#7768=VERTEX_POINT('',#27234);
#7769=VERTEX_POINT('',#27236);
#7770=VERTEX_POINT('',#27240);
#7771=VERTEX_POINT('',#27242);
#7772=VERTEX_POINT('',#27247);
#7773=VERTEX_POINT('',#27251);
#7774=VERTEX_POINT('',#27255);
#7775=VERTEX_POINT('',#27259);
#7776=VERTEX_POINT('',#27261);
#7777=VERTEX_POINT('',#27263);
#7778=VERTEX_POINT('',#27266);
#7779=VERTEX_POINT('',#27270);
#7780=VERTEX_POINT('',#27272);
#7781=VERTEX_POINT('',#27276);
#7782=VERTEX_POINT('',#27278);
#9646=EDGE_CURVE('',#7633,#7634,#1255,.T.);
#9647=EDGE_CURVE('',#7635,#7633,#4229,.T.);
#9648=EDGE_CURVE('',#7636,#7635,#1256,.T.);
#9649=EDGE_CURVE('',#7634,#7636,#4230,.T.);
#9650=EDGE_CURVE('',#7637,#7638,#1257,.T.);
#9651=EDGE_CURVE('',#7639,#7637,#4231,.T.);
#9652=EDGE_CURVE('',#7640,#7639,#1258,.T.);
#9653=EDGE_CURVE('',#7638,#7640,#4232,.T.);
#9654=EDGE_CURVE('',#7641,#7642,#1259,.T.);
#9655=EDGE_CURVE('',#7643,#7641,#4233,.T.);
#9656=EDGE_CURVE('',#7644,#7643,#1260,.T.);
#9657=EDGE_CURVE('',#7642,#7644,#4234,.T.);
#9658=EDGE_CURVE('',#7645,#7646,#1261,.T.);
#9659=EDGE_CURVE('',#7647,#7645,#4235,.T.);
#9660=EDGE_CURVE('',#7648,#7647,#1262,.T.);
#9661=EDGE_CURVE('',#7646,#7648,#4236,.T.);
#9662=EDGE_CURVE('',#7649,#7650,#1263,.T.);
#9663=EDGE_CURVE('',#7651,#7649,#4237,.T.);
#9664=EDGE_CURVE('',#7652,#7651,#1264,.T.);
#9665=EDGE_CURVE('',#7650,#7652,#4238,.T.);
#9666=EDGE_CURVE('',#7653,#7654,#1265,.T.);
#9667=EDGE_CURVE('',#7655,#7653,#4239,.T.);
#9668=EDGE_CURVE('',#7656,#7655,#1266,.T.);
#9669=EDGE_CURVE('',#7654,#7656,#4240,.T.);
#9670=EDGE_CURVE('',#7657,#7658,#1267,.T.);
#9671=EDGE_CURVE('',#7658,#7657,#1268,.T.);
#9672=EDGE_CURVE('',#7658,#7659,#4241,.T.);
#9673=EDGE_CURVE('',#7659,#7659,#1269,.T.);
#9674=EDGE_CURVE('',#7660,#7661,#1270,.T.);
#9675=EDGE_CURVE('',#7661,#7660,#1271,.T.);
#9676=EDGE_CURVE('',#7661,#7662,#4242,.T.);
#9677=EDGE_CURVE('',#7662,#7662,#1272,.T.);
#9678=EDGE_CURVE('',#7663,#7664,#1273,.T.);
#9679=EDGE_CURVE('',#7664,#7663,#1274,.T.);
#9680=EDGE_CURVE('',#7664,#7665,#4243,.T.);
#9681=EDGE_CURVE('',#7665,#7665,#1275,.T.);
#9682=EDGE_CURVE('',#7666,#7667,#1276,.T.);
#9683=EDGE_CURVE('',#7667,#7666,#1277,.T.);
#9684=EDGE_CURVE('',#7667,#7668,#4244,.T.);
#9685=EDGE_CURVE('',#7668,#7668,#1278,.T.);
#9686=EDGE_CURVE('',#7669,#7670,#1279,.T.);
#9687=EDGE_CURVE('',#7670,#7669,#1280,.T.);
#9688=EDGE_CURVE('',#7670,#7671,#4245,.T.);
#9689=EDGE_CURVE('',#7671,#7671,#1281,.T.);
#9690=EDGE_CURVE('',#7672,#7673,#1282,.T.);
#9691=EDGE_CURVE('',#7673,#7672,#1283,.T.);
#9692=EDGE_CURVE('',#7673,#7674,#4246,.T.);
#9693=EDGE_CURVE('',#7674,#7674,#1284,.T.);
#9694=EDGE_CURVE('',#7675,#7676,#1285,.T.);
#9695=EDGE_CURVE('',#7676,#7675,#1286,.T.);
#9696=EDGE_CURVE('',#7676,#7677,#4247,.T.);
#9697=EDGE_CURVE('',#7677,#7677,#1287,.T.);
#9698=EDGE_CURVE('',#7678,#7679,#1288,.T.);
#9699=EDGE_CURVE('',#7679,#7678,#1289,.T.);
#9700=EDGE_CURVE('',#7679,#7680,#4248,.T.);
#9701=EDGE_CURVE('',#7680,#7680,#1290,.T.);
#9702=EDGE_CURVE('',#7681,#7682,#1291,.T.);
#9703=EDGE_CURVE('',#7682,#7681,#1292,.T.);
#9704=EDGE_CURVE('',#7682,#7683,#4249,.T.);
#9705=EDGE_CURVE('',#7683,#7683,#1293,.T.);
#9706=EDGE_CURVE('',#7684,#7685,#1294,.T.);
#9707=EDGE_CURVE('',#7685,#7684,#1295,.T.);
#9708=EDGE_CURVE('',#7685,#7686,#4250,.T.);
#9709=EDGE_CURVE('',#7686,#7686,#1296,.T.);
#9710=EDGE_CURVE('',#7687,#7688,#1297,.T.);
#9711=EDGE_CURVE('',#7688,#7687,#1298,.T.);
#9712=EDGE_CURVE('',#7688,#7689,#4251,.T.);
#9713=EDGE_CURVE('',#7689,#7689,#1299,.T.);
#9714=EDGE_CURVE('',#7690,#7691,#1300,.T.);
#9715=EDGE_CURVE('',#7691,#7690,#1301,.T.);
#9716=EDGE_CURVE('',#7691,#7692,#4252,.T.);
#9717=EDGE_CURVE('',#7692,#7692,#1302,.T.);
#9718=EDGE_CURVE('',#7693,#7694,#1303,.T.);
#9719=EDGE_CURVE('',#7694,#7693,#1304,.T.);
#9720=EDGE_CURVE('',#7694,#7695,#4253,.T.);
#9721=EDGE_CURVE('',#7695,#7695,#1305,.T.);
#9722=EDGE_CURVE('',#7696,#7697,#4254,.T.);
#9723=EDGE_CURVE('',#7697,#7698,#4255,.T.);
#9724=EDGE_CURVE('',#7698,#7699,#4256,.T.);
#9725=EDGE_CURVE('',#7699,#7696,#4257,.T.);
#9726=EDGE_CURVE('',#7700,#7701,#1306,.T.);
#9727=EDGE_CURVE('',#7702,#7701,#4258,.T.);
#9728=EDGE_CURVE('',#7703,#7702,#4259,.T.);
#9729=EDGE_CURVE('',#7704,#7703,#1307,.T.);
#9730=EDGE_CURVE('',#7705,#7704,#4260,.T.);
#9731=EDGE_CURVE('',#7706,#7705,#1308,.T.);
#9732=EDGE_CURVE('',#7706,#7707,#4261,.T.);
#9733=EDGE_CURVE('',#7707,#7708,#4262,.T.);
#9734=EDGE_CURVE('',#7708,#7700,#4263,.T.);
#9735=EDGE_CURVE('',#7709,#7710,#4264,.T.);
#9736=EDGE_CURVE('',#7710,#7711,#4265,.T.);
#9737=EDGE_CURVE('',#7711,#7712,#4266,.T.);
#9738=EDGE_CURVE('',#7712,#7709,#4267,.T.);
#9739=EDGE_CURVE('',#7713,#7714,#4268,.T.);
#9740=EDGE_CURVE('',#7711,#7714,#4269,.T.);
#9741=EDGE_CURVE('',#7715,#7710,#4270,.T.);
#9742=EDGE_CURVE('',#7715,#7713,#4271,.T.);
#9743=EDGE_CURVE('',#7714,#7716,#4272,.T.);
#9744=EDGE_CURVE('',#7712,#7716,#4273,.T.);
#9745=EDGE_CURVE('',#7716,#7717,#4274,.T.);
#9746=EDGE_CURVE('',#7718,#7717,#4275,.T.);
#9747=EDGE_CURVE('',#7709,#7718,#4276,.T.);
#9748=EDGE_CURVE('',#7704,#7719,#4277,.T.);
#9749=EDGE_CURVE('',#7720,#7703,#4278,.T.);
#9750=EDGE_CURVE('',#7719,#7720,#1309,.T.);
#9751=EDGE_CURVE('',#7706,#7709,#4279,.T.);
#9752=EDGE_CURVE('',#7721,#7705,#4280,.T.);
#9753=EDGE_CURVE('',#7722,#7721,#1310,.T.);
#9754=EDGE_CURVE('',#7710,#7722,#4281,.T.);
#9755=EDGE_CURVE('',#7723,#7724,#1311,.T.);
#9756=EDGE_CURVE('',#7725,#7723,#4282,.T.);
#9757=EDGE_CURVE('',#7726,#7725,#1312,.T.);
#9758=EDGE_CURVE('',#7724,#7726,#4283,.T.);
#9759=EDGE_CURVE('',#7716,#7700,#4284,.T.);
#9760=EDGE_CURVE('',#7727,#7714,#4285,.T.);
#9761=EDGE_CURVE('',#7728,#7727,#1313,.T.);
#9762=EDGE_CURVE('',#7701,#7728,#4286,.T.);
#9763=EDGE_CURVE('',#7728,#7729,#4287,.T.);
#9764=EDGE_CURVE('',#7730,#7727,#4288,.T.);
#9765=EDGE_CURVE('',#7731,#7730,#4289,.T.);
#9766=EDGE_CURVE('',#7722,#7731,#4290,.T.);
#9767=EDGE_CURVE('',#7732,#7721,#4291,.T.);
#9768=EDGE_CURVE('',#7729,#7732,#4292,.T.);
#9769=EDGE_CURVE('',#7731,#7715,#4293,.T.);
#9770=EDGE_CURVE('',#7730,#7713,#4294,.T.);
#9771=EDGE_CURVE('',#7647,#7636,#4295,.T.);
#9772=EDGE_CURVE('',#7645,#7634,#4296,.T.);
#9773=EDGE_CURVE('',#7641,#7646,#4297,.T.);
#9774=EDGE_CURVE('',#7643,#7648,#4298,.T.);
#9775=EDGE_CURVE('',#7637,#7642,#4299,.T.);
#9776=EDGE_CURVE('',#7639,#7644,#4300,.T.);
#9777=EDGE_CURVE('',#7633,#7638,#4301,.T.);
#9778=EDGE_CURVE('',#7635,#7640,#4302,.T.);
#9779=EDGE_CURVE('',#7693,#7733,#4303,.T.);
#9780=EDGE_CURVE('',#7733,#7733,#1314,.T.);
#9781=EDGE_CURVE('',#7734,#7734,#1315,.T.);
#9782=EDGE_CURVE('',#7734,#7735,#4304,.T.);
#9783=EDGE_CURVE('',#7735,#7735,#1316,.T.);
#9784=EDGE_CURVE('',#7687,#7736,#4305,.T.);
#9785=EDGE_CURVE('',#7736,#7736,#1317,.T.);
#9786=EDGE_CURVE('',#7675,#7737,#4306,.T.);
#9787=EDGE_CURVE('',#7737,#7737,#1318,.T.);
#9788=EDGE_CURVE('',#7690,#7738,#4307,.T.);
#9789=EDGE_CURVE('',#7738,#7738,#1319,.T.);
#9790=EDGE_CURVE('',#7739,#7739,#1320,.T.);
#9791=EDGE_CURVE('',#7739,#7740,#4308,.T.);
#9792=EDGE_CURVE('',#7740,#7740,#1321,.T.);
#9793=EDGE_CURVE('',#7741,#7741,#1322,.T.);
#9794=EDGE_CURVE('',#7741,#7742,#4309,.T.);
#9795=EDGE_CURVE('',#7742,#7742,#1323,.T.);
#9796=EDGE_CURVE('',#7684,#7743,#4310,.T.);
#9797=EDGE_CURVE('',#7743,#7743,#1324,.T.);
#9798=EDGE_CURVE('',#7672,#7744,#4311,.T.);
#9799=EDGE_CURVE('',#7744,#7744,#1325,.T.);
#9800=EDGE_CURVE('',#7681,#7745,#4312,.T.);
#9801=EDGE_CURVE('',#7745,#7745,#1326,.T.);
#9802=EDGE_CURVE('',#7678,#7746,#4313,.T.);
#9803=EDGE_CURVE('',#7746,#7746,#1327,.T.);
#9804=EDGE_CURVE('',#7669,#7747,#4314,.T.);
#9805=EDGE_CURVE('',#7747,#7747,#1328,.T.);
#9806=EDGE_CURVE('',#7666,#7748,#4315,.T.);
#9807=EDGE_CURVE('',#7748,#7748,#1329,.T.);
#9808=EDGE_CURVE('',#7663,#7749,#4316,.T.);
#9809=EDGE_CURVE('',#7749,#7749,#1330,.T.);
#9810=EDGE_CURVE('',#7657,#7750,#4317,.T.);
#9811=EDGE_CURVE('',#7750,#7750,#1331,.T.);
#9812=EDGE_CURVE('',#7660,#7751,#4318,.T.);
#9813=EDGE_CURVE('',#7751,#7751,#1332,.T.);
#9814=EDGE_CURVE('',#7752,#7753,#4319,.T.);
#9815=EDGE_CURVE('',#7754,#7753,#4320,.T.);
#9816=EDGE_CURVE('',#7755,#7754,#4321,.T.);
#9817=EDGE_CURVE('',#7755,#7752,#4322,.T.);
#9818=EDGE_CURVE('',#7756,#7752,#4323,.T.);
#9819=EDGE_CURVE('',#7757,#7755,#4324,.T.);
#9820=EDGE_CURVE('',#7757,#7756,#4325,.T.);
#9821=EDGE_CURVE('',#7650,#7757,#4326,.T.);
#9822=EDGE_CURVE('',#7652,#7756,#4327,.T.);
#9823=EDGE_CURVE('',#7758,#7651,#4328,.T.);
#9824=EDGE_CURVE('',#7759,#7649,#4329,.T.);
#9825=EDGE_CURVE('',#7759,#7758,#4330,.T.);
#9826=EDGE_CURVE('',#7760,#7758,#1333,.T.);
#9827=EDGE_CURVE('',#7761,#7759,#1334,.T.);
#9828=EDGE_CURVE('',#7761,#7760,#4331,.T.);
#9829=EDGE_CURVE('',#7654,#7761,#4332,.T.);
#9830=EDGE_CURVE('',#7656,#7760,#4333,.T.);
#9831=EDGE_CURVE('',#7762,#7655,#4334,.T.);
#9832=EDGE_CURVE('',#7763,#7653,#4335,.T.);
#9833=EDGE_CURVE('',#7763,#7762,#4336,.T.);
#9834=EDGE_CURVE('',#7764,#7762,#1335,.T.);
#9835=EDGE_CURVE('',#7765,#7763,#1336,.T.);
#9836=EDGE_CURVE('',#7765,#7764,#4337,.T.);
#9837=EDGE_CURVE('',#7766,#7764,#4338,.T.);
#9838=EDGE_CURVE('',#7767,#7765,#4339,.T.);
#9839=EDGE_CURVE('',#7767,#7766,#4340,.T.);
#9840=EDGE_CURVE('',#7768,#7766,#1337,.T.);
#9841=EDGE_CURVE('',#7769,#7767,#1338,.T.);
#9842=EDGE_CURVE('',#7769,#7768,#4341,.T.);
#9843=EDGE_CURVE('',#7770,#7768,#4342,.T.);
#9844=EDGE_CURVE('',#7771,#7769,#4343,.T.);
#9845=EDGE_CURVE('',#7771,#7770,#4344,.T.);
#9846=EDGE_CURVE('',#7725,#7697,#4345,.T.);
#9847=EDGE_CURVE('',#7723,#7772,#4346,.T.);
#9848=EDGE_CURVE('',#7702,#7772,#4347,.T.);
#9849=EDGE_CURVE('',#7729,#7770,#4348,.T.);
#9850=EDGE_CURVE('',#7773,#7771,#4349,.T.);
#9851=EDGE_CURVE('',#7773,#7698,#4350,.T.);
#9852=EDGE_CURVE('',#7774,#7699,#4351,.T.);
#9853=EDGE_CURVE('',#7774,#7773,#4352,.T.);
#9854=EDGE_CURVE('',#7775,#7696,#4353,.T.);
#9855=EDGE_CURVE('',#7776,#7774,#4354,.T.);
#9856=EDGE_CURVE('',#7776,#7777,#4355,.T.);
#9857=EDGE_CURVE('',#7732,#7777,#4356,.T.);
#9858=EDGE_CURVE('',#7778,#7719,#4357,.T.);
#9859=EDGE_CURVE('',#7775,#7778,#4358,.T.);
#9860=EDGE_CURVE('',#7779,#7777,#4359,.T.);
#9861=EDGE_CURVE('',#7780,#7776,#4360,.T.);
#9862=EDGE_CURVE('',#7780,#7779,#4361,.T.);
#9863=EDGE_CURVE('',#7781,#7779,#4362,.T.);
#9864=EDGE_CURVE('',#7782,#7780,#4363,.T.);
#9865=EDGE_CURVE('',#7782,#7781,#4364,.T.);
#9866=EDGE_CURVE('',#7720,#7781,#4365,.T.);
#9867=EDGE_CURVE('',#7778,#7782,#4366,.T.);
#9868=EDGE_CURVE('',#7726,#7775,#4367,.T.);
#9869=EDGE_CURVE('',#7753,#7772,#4368,.T.);
#9870=EDGE_CURVE('',#7754,#7724,#4369,.T.);
#9871=EDGE_CURVE('',#7718,#7707,#4370,.T.);
#9872=EDGE_CURVE('',#7717,#7708,#4371,.T.);
#13188=ORIENTED_EDGE('',*,*,#9646,.F.);
#13189=ORIENTED_EDGE('',*,*,#9647,.F.);
#13190=ORIENTED_EDGE('',*,*,#9648,.F.);
#13191=ORIENTED_EDGE('',*,*,#9649,.F.);
#13192=ORIENTED_EDGE('',*,*,#9650,.F.);
#13193=ORIENTED_EDGE('',*,*,#9651,.F.);
#13194=ORIENTED_EDGE('',*,*,#9652,.F.);
#13195=ORIENTED_EDGE('',*,*,#9653,.F.);
#13196=ORIENTED_EDGE('',*,*,#9654,.F.);
#13197=ORIENTED_EDGE('',*,*,#9655,.F.);
#13198=ORIENTED_EDGE('',*,*,#9656,.F.);
#13199=ORIENTED_EDGE('',*,*,#9657,.F.);
#13200=ORIENTED_EDGE('',*,*,#9658,.F.);
#13201=ORIENTED_EDGE('',*,*,#9659,.F.);
#13202=ORIENTED_EDGE('',*,*,#9660,.F.);
#13203=ORIENTED_EDGE('',*,*,#9661,.F.);
#13204=ORIENTED_EDGE('',*,*,#9662,.F.);
#13205=ORIENTED_EDGE('',*,*,#9663,.F.);
#13206=ORIENTED_EDGE('',*,*,#9664,.F.);
#13207=ORIENTED_EDGE('',*,*,#9665,.F.);
#13208=ORIENTED_EDGE('',*,*,#9666,.F.);
#13209=ORIENTED_EDGE('',*,*,#9667,.F.);
#13210=ORIENTED_EDGE('',*,*,#9668,.F.);
#13211=ORIENTED_EDGE('',*,*,#9669,.F.);
#13212=ORIENTED_EDGE('',*,*,#9670,.F.);
#13213=ORIENTED_EDGE('',*,*,#9671,.F.);
#13214=ORIENTED_EDGE('',*,*,#9672,.T.);
#13215=ORIENTED_EDGE('',*,*,#9673,.F.);
#13216=ORIENTED_EDGE('',*,*,#9672,.F.);
#13217=ORIENTED_EDGE('',*,*,#9674,.F.);
#13218=ORIENTED_EDGE('',*,*,#9675,.F.);
#13219=ORIENTED_EDGE('',*,*,#9676,.T.);
#13220=ORIENTED_EDGE('',*,*,#9677,.F.);
#13221=ORIENTED_EDGE('',*,*,#9676,.F.);
#13222=ORIENTED_EDGE('',*,*,#9678,.F.);
#13223=ORIENTED_EDGE('',*,*,#9679,.F.);
#13224=ORIENTED_EDGE('',*,*,#9680,.T.);
#13225=ORIENTED_EDGE('',*,*,#9681,.F.);
#13226=ORIENTED_EDGE('',*,*,#9680,.F.);
#13227=ORIENTED_EDGE('',*,*,#9682,.F.);
#13228=ORIENTED_EDGE('',*,*,#9683,.F.);
#13229=ORIENTED_EDGE('',*,*,#9684,.T.);
#13230=ORIENTED_EDGE('',*,*,#9685,.F.);
#13231=ORIENTED_EDGE('',*,*,#9684,.F.);
#13232=ORIENTED_EDGE('',*,*,#9686,.F.);
#13233=ORIENTED_EDGE('',*,*,#9687,.F.);
#13234=ORIENTED_EDGE('',*,*,#9688,.T.);
#13235=ORIENTED_EDGE('',*,*,#9689,.F.);
#13236=ORIENTED_EDGE('',*,*,#9688,.F.);
#13237=ORIENTED_EDGE('',*,*,#9690,.F.);
#13238=ORIENTED_EDGE('',*,*,#9691,.F.);
#13239=ORIENTED_EDGE('',*,*,#9692,.T.);
#13240=ORIENTED_EDGE('',*,*,#9693,.F.);
#13241=ORIENTED_EDGE('',*,*,#9692,.F.);
#13242=ORIENTED_EDGE('',*,*,#9694,.F.);
#13243=ORIENTED_EDGE('',*,*,#9695,.F.);
#13244=ORIENTED_EDGE('',*,*,#9696,.T.);
#13245=ORIENTED_EDGE('',*,*,#9697,.F.);
#13246=ORIENTED_EDGE('',*,*,#9696,.F.);
#13247=ORIENTED_EDGE('',*,*,#9698,.F.);
#13248=ORIENTED_EDGE('',*,*,#9699,.F.);
#13249=ORIENTED_EDGE('',*,*,#9700,.T.);
#13250=ORIENTED_EDGE('',*,*,#9701,.F.);
#13251=ORIENTED_EDGE('',*,*,#9700,.F.);
#13252=ORIENTED_EDGE('',*,*,#9702,.F.);
#13253=ORIENTED_EDGE('',*,*,#9703,.F.);
#13254=ORIENTED_EDGE('',*,*,#9704,.T.);
#13255=ORIENTED_EDGE('',*,*,#9705,.F.);
#13256=ORIENTED_EDGE('',*,*,#9704,.F.);
#13257=ORIENTED_EDGE('',*,*,#9706,.F.);
#13258=ORIENTED_EDGE('',*,*,#9707,.F.);
#13259=ORIENTED_EDGE('',*,*,#9708,.T.);
#13260=ORIENTED_EDGE('',*,*,#9709,.F.);
#13261=ORIENTED_EDGE('',*,*,#9708,.F.);
#13262=ORIENTED_EDGE('',*,*,#9710,.F.);
#13263=ORIENTED_EDGE('',*,*,#9711,.F.);
#13264=ORIENTED_EDGE('',*,*,#9712,.T.);
#13265=ORIENTED_EDGE('',*,*,#9713,.F.);
#13266=ORIENTED_EDGE('',*,*,#9712,.F.);
#13267=ORIENTED_EDGE('',*,*,#9714,.F.);
#13268=ORIENTED_EDGE('',*,*,#9715,.F.);
#13269=ORIENTED_EDGE('',*,*,#9716,.T.);
#13270=ORIENTED_EDGE('',*,*,#9717,.F.);
#13271=ORIENTED_EDGE('',*,*,#9716,.F.);
#13272=ORIENTED_EDGE('',*,*,#9718,.F.);
#13273=ORIENTED_EDGE('',*,*,#9719,.F.);
#13274=ORIENTED_EDGE('',*,*,#9720,.T.);
#13275=ORIENTED_EDGE('',*,*,#9721,.F.);
#13276=ORIENTED_EDGE('',*,*,#9720,.F.);
#13277=ORIENTED_EDGE('',*,*,#9722,.T.);
#13278=ORIENTED_EDGE('',*,*,#9723,.T.);
#13279=ORIENTED_EDGE('',*,*,#9724,.T.);
#13280=ORIENTED_EDGE('',*,*,#9725,.T.);
#13281=ORIENTED_EDGE('',*,*,#9726,.T.);
#13282=ORIENTED_EDGE('',*,*,#9727,.F.);
#13283=ORIENTED_EDGE('',*,*,#9728,.F.);
#13284=ORIENTED_EDGE('',*,*,#9729,.F.);
#13285=ORIENTED_EDGE('',*,*,#9730,.F.);
#13286=ORIENTED_EDGE('',*,*,#9731,.F.);
#13287=ORIENTED_EDGE('',*,*,#9732,.T.);
#13288=ORIENTED_EDGE('',*,*,#9733,.T.);
#13289=ORIENTED_EDGE('',*,*,#9734,.T.);
#13290=ORIENTED_EDGE('',*,*,#9735,.T.);
#13291=ORIENTED_EDGE('',*,*,#9736,.T.);
#13292=ORIENTED_EDGE('',*,*,#9737,.T.);
#13293=ORIENTED_EDGE('',*,*,#9738,.T.);
#13294=ORIENTED_EDGE('',*,*,#9739,.T.);
#13295=ORIENTED_EDGE('',*,*,#9740,.F.);
#13296=ORIENTED_EDGE('',*,*,#9736,.F.);
#13297=ORIENTED_EDGE('',*,*,#9741,.F.);
#13298=ORIENTED_EDGE('',*,*,#9742,.T.);
#13299=ORIENTED_EDGE('',*,*,#9743,.T.);
#13300=ORIENTED_EDGE('',*,*,#9744,.F.);
#13301=ORIENTED_EDGE('',*,*,#9737,.F.);
#13302=ORIENTED_EDGE('',*,*,#9740,.T.);
#13303=ORIENTED_EDGE('',*,*,#9745,.T.);
#13304=ORIENTED_EDGE('',*,*,#9746,.F.);
#13305=ORIENTED_EDGE('',*,*,#9747,.F.);
#13306=ORIENTED_EDGE('',*,*,#9738,.F.);
#13307=ORIENTED_EDGE('',*,*,#9744,.T.);
#13308=ORIENTED_EDGE('',*,*,#9748,.F.);
#13309=ORIENTED_EDGE('',*,*,#9729,.T.);
#13310=ORIENTED_EDGE('',*,*,#9749,.F.);
#13311=ORIENTED_EDGE('',*,*,#9750,.F.);
#13312=ORIENTED_EDGE('',*,*,#9751,.F.);
#13313=ORIENTED_EDGE('',*,*,#9731,.T.);
#13314=ORIENTED_EDGE('',*,*,#9752,.F.);
#13315=ORIENTED_EDGE('',*,*,#9753,.F.);
#13316=ORIENTED_EDGE('',*,*,#9754,.F.);
#13317=ORIENTED_EDGE('',*,*,#9735,.F.);
#13318=ORIENTED_EDGE('',*,*,#9755,.F.);
#13319=ORIENTED_EDGE('',*,*,#9756,.F.);
#13320=ORIENTED_EDGE('',*,*,#9757,.F.);
#13321=ORIENTED_EDGE('',*,*,#9758,.F.);
#13322=ORIENTED_EDGE('',*,*,#9726,.F.);
#13323=ORIENTED_EDGE('',*,*,#9759,.F.);
#13324=ORIENTED_EDGE('',*,*,#9743,.F.);
#13325=ORIENTED_EDGE('',*,*,#9760,.F.);
#13326=ORIENTED_EDGE('',*,*,#9761,.F.);
#13327=ORIENTED_EDGE('',*,*,#9762,.F.);
#13328=ORIENTED_EDGE('',*,*,#9763,.F.);
#13329=ORIENTED_EDGE('',*,*,#9761,.T.);
#13330=ORIENTED_EDGE('',*,*,#9764,.F.);
#13331=ORIENTED_EDGE('',*,*,#9765,.F.);
#13332=ORIENTED_EDGE('',*,*,#9766,.F.);
#13333=ORIENTED_EDGE('',*,*,#9753,.T.);
#13334=ORIENTED_EDGE('',*,*,#9767,.F.);
#13335=ORIENTED_EDGE('',*,*,#9768,.F.);
#13336=ORIENTED_EDGE('',*,*,#9741,.T.);
#13337=ORIENTED_EDGE('',*,*,#9754,.T.);
#13338=ORIENTED_EDGE('',*,*,#9766,.T.);
#13339=ORIENTED_EDGE('',*,*,#9769,.T.);
#13340=ORIENTED_EDGE('',*,*,#9742,.F.);
#13341=ORIENTED_EDGE('',*,*,#9769,.F.);
#13342=ORIENTED_EDGE('',*,*,#9765,.T.);
#13343=ORIENTED_EDGE('',*,*,#9770,.T.);
#13344=ORIENTED_EDGE('',*,*,#9739,.F.);
#13345=ORIENTED_EDGE('',*,*,#9770,.F.);
#13346=ORIENTED_EDGE('',*,*,#9764,.T.);
#13347=ORIENTED_EDGE('',*,*,#9760,.T.);
#13348=ORIENTED_EDGE('',*,*,#9771,.F.);
#13349=ORIENTED_EDGE('',*,*,#9659,.T.);
#13350=ORIENTED_EDGE('',*,*,#9772,.T.);
#13351=ORIENTED_EDGE('',*,*,#9649,.T.);
#13352=ORIENTED_EDGE('',*,*,#9773,.T.);
#13353=ORIENTED_EDGE('',*,*,#9661,.T.);
#13354=ORIENTED_EDGE('',*,*,#9774,.F.);
#13355=ORIENTED_EDGE('',*,*,#9655,.T.);
#13356=ORIENTED_EDGE('',*,*,#9775,.T.);
#13357=ORIENTED_EDGE('',*,*,#9657,.T.);
#13358=ORIENTED_EDGE('',*,*,#9776,.F.);
#13359=ORIENTED_EDGE('',*,*,#9651,.T.);
#13360=ORIENTED_EDGE('',*,*,#9777,.T.);
#13361=ORIENTED_EDGE('',*,*,#9653,.T.);
#13362=ORIENTED_EDGE('',*,*,#9778,.F.);
#13363=ORIENTED_EDGE('',*,*,#9647,.T.);
#13364=ORIENTED_EDGE('',*,*,#9718,.T.);
#13365=ORIENTED_EDGE('',*,*,#9719,.T.);
#13366=ORIENTED_EDGE('',*,*,#9779,.T.);
#13367=ORIENTED_EDGE('',*,*,#9780,.F.);
#13368=ORIENTED_EDGE('',*,*,#9779,.F.);
#13369=ORIENTED_EDGE('',*,*,#9781,.T.);
#13370=ORIENTED_EDGE('',*,*,#9782,.T.);
#13371=ORIENTED_EDGE('',*,*,#9783,.F.);
#13372=ORIENTED_EDGE('',*,*,#9782,.F.);
#13373=ORIENTED_EDGE('',*,*,#9710,.T.);
#13374=ORIENTED_EDGE('',*,*,#9711,.T.);
#13375=ORIENTED_EDGE('',*,*,#9784,.T.);
#13376=ORIENTED_EDGE('',*,*,#9785,.F.);
#13377=ORIENTED_EDGE('',*,*,#9784,.F.);
#13378=ORIENTED_EDGE('',*,*,#9694,.T.);
#13379=ORIENTED_EDGE('',*,*,#9695,.T.);
#13380=ORIENTED_EDGE('',*,*,#9786,.T.);
#13381=ORIENTED_EDGE('',*,*,#9787,.F.);
#13382=ORIENTED_EDGE('',*,*,#9786,.F.);
#13383=ORIENTED_EDGE('',*,*,#9714,.T.);
#13384=ORIENTED_EDGE('',*,*,#9715,.T.);
#13385=ORIENTED_EDGE('',*,*,#9788,.T.);
#13386=ORIENTED_EDGE('',*,*,#9789,.F.);
#13387=ORIENTED_EDGE('',*,*,#9788,.F.);
#13388=ORIENTED_EDGE('',*,*,#9790,.T.);
#13389=ORIENTED_EDGE('',*,*,#9791,.T.);
#13390=ORIENTED_EDGE('',*,*,#9792,.F.);
#13391=ORIENTED_EDGE('',*,*,#9791,.F.);
#13392=ORIENTED_EDGE('',*,*,#9793,.T.);
#13393=ORIENTED_EDGE('',*,*,#9794,.T.);
#13394=ORIENTED_EDGE('',*,*,#9795,.F.);
#13395=ORIENTED_EDGE('',*,*,#9794,.F.);
#13396=ORIENTED_EDGE('',*,*,#9706,.T.);
#13397=ORIENTED_EDGE('',*,*,#9707,.T.);
#13398=ORIENTED_EDGE('',*,*,#9796,.T.);
#13399=ORIENTED_EDGE('',*,*,#9797,.F.);
#13400=ORIENTED_EDGE('',*,*,#9796,.F.);
#13401=ORIENTED_EDGE('',*,*,#9690,.T.);
#13402=ORIENTED_EDGE('',*,*,#9691,.T.);
#13403=ORIENTED_EDGE('',*,*,#9798,.T.);
#13404=ORIENTED_EDGE('',*,*,#9799,.F.);
#13405=ORIENTED_EDGE('',*,*,#9798,.F.);
#13406=ORIENTED_EDGE('',*,*,#9702,.T.);
#13407=ORIENTED_EDGE('',*,*,#9703,.T.);
#13408=ORIENTED_EDGE('',*,*,#9800,.T.);
#13409=ORIENTED_EDGE('',*,*,#9801,.F.);
#13410=ORIENTED_EDGE('',*,*,#9800,.F.);
#13411=ORIENTED_EDGE('',*,*,#9698,.T.);
#13412=ORIENTED_EDGE('',*,*,#9699,.T.);
#13413=ORIENTED_EDGE('',*,*,#9802,.T.);
#13414=ORIENTED_EDGE('',*,*,#9803,.F.);
#13415=ORIENTED_EDGE('',*,*,#9802,.F.);
#13416=ORIENTED_EDGE('',*,*,#9686,.T.);
#13417=ORIENTED_EDGE('',*,*,#9687,.T.);
#13418=ORIENTED_EDGE('',*,*,#9804,.T.);
#13419=ORIENTED_EDGE('',*,*,#9805,.F.);
#13420=ORIENTED_EDGE('',*,*,#9804,.F.);
#13421=ORIENTED_EDGE('',*,*,#9682,.T.);
#13422=ORIENTED_EDGE('',*,*,#9683,.T.);
#13423=ORIENTED_EDGE('',*,*,#9806,.T.);
#13424=ORIENTED_EDGE('',*,*,#9807,.F.);
#13425=ORIENTED_EDGE('',*,*,#9806,.F.);
#13426=ORIENTED_EDGE('',*,*,#9678,.T.);
#13427=ORIENTED_EDGE('',*,*,#9679,.T.);
#13428=ORIENTED_EDGE('',*,*,#9808,.T.);
#13429=ORIENTED_EDGE('',*,*,#9809,.F.);
#13430=ORIENTED_EDGE('',*,*,#9808,.F.);
#13431=ORIENTED_EDGE('',*,*,#9670,.T.);
#13432=ORIENTED_EDGE('',*,*,#9671,.T.);
#13433=ORIENTED_EDGE('',*,*,#9810,.T.);
#13434=ORIENTED_EDGE('',*,*,#9811,.F.);
#13435=ORIENTED_EDGE('',*,*,#9810,.F.);
#13436=ORIENTED_EDGE('',*,*,#9674,.T.);
#13437=ORIENTED_EDGE('',*,*,#9675,.T.);
#13438=ORIENTED_EDGE('',*,*,#9812,.T.);
#13439=ORIENTED_EDGE('',*,*,#9813,.F.);
#13440=ORIENTED_EDGE('',*,*,#9812,.F.);
#13441=ORIENTED_EDGE('',*,*,#9814,.T.);
#13442=ORIENTED_EDGE('',*,*,#9815,.F.);
#13443=ORIENTED_EDGE('',*,*,#9816,.F.);
#13444=ORIENTED_EDGE('',*,*,#9817,.T.);
#13445=ORIENTED_EDGE('',*,*,#9818,.T.);
#13446=ORIENTED_EDGE('',*,*,#9817,.F.);
#13447=ORIENTED_EDGE('',*,*,#9819,.F.);
#13448=ORIENTED_EDGE('',*,*,#9820,.T.);
#13449=ORIENTED_EDGE('',*,*,#9821,.F.);
#13450=ORIENTED_EDGE('',*,*,#9665,.T.);
#13451=ORIENTED_EDGE('',*,*,#9822,.T.);
#13452=ORIENTED_EDGE('',*,*,#9820,.F.);
#13453=ORIENTED_EDGE('',*,*,#9823,.T.);
#13454=ORIENTED_EDGE('',*,*,#9663,.T.);
#13455=ORIENTED_EDGE('',*,*,#9824,.F.);
#13456=ORIENTED_EDGE('',*,*,#9825,.T.);
#13457=ORIENTED_EDGE('',*,*,#9826,.T.);
#13458=ORIENTED_EDGE('',*,*,#9825,.F.);
#13459=ORIENTED_EDGE('',*,*,#9827,.F.);
#13460=ORIENTED_EDGE('',*,*,#9828,.T.);
#13461=ORIENTED_EDGE('',*,*,#9829,.F.);
#13462=ORIENTED_EDGE('',*,*,#9669,.T.);
#13463=ORIENTED_EDGE('',*,*,#9830,.T.);
#13464=ORIENTED_EDGE('',*,*,#9828,.F.);
#13465=ORIENTED_EDGE('',*,*,#9831,.T.);
#13466=ORIENTED_EDGE('',*,*,#9667,.T.);
#13467=ORIENTED_EDGE('',*,*,#9832,.F.);
#13468=ORIENTED_EDGE('',*,*,#9833,.T.);
#13469=ORIENTED_EDGE('',*,*,#9834,.T.);
#13470=ORIENTED_EDGE('',*,*,#9833,.F.);
#13471=ORIENTED_EDGE('',*,*,#9835,.F.);
#13472=ORIENTED_EDGE('',*,*,#9836,.T.);
#13473=ORIENTED_EDGE('',*,*,#9837,.T.);
#13474=ORIENTED_EDGE('',*,*,#9836,.F.);
#13475=ORIENTED_EDGE('',*,*,#9838,.F.);
#13476=ORIENTED_EDGE('',*,*,#9839,.T.);
#13477=ORIENTED_EDGE('',*,*,#9840,.T.);
#13478=ORIENTED_EDGE('',*,*,#9839,.F.);
#13479=ORIENTED_EDGE('',*,*,#9841,.F.);
#13480=ORIENTED_EDGE('',*,*,#9842,.T.);
#13481=ORIENTED_EDGE('',*,*,#9843,.T.);
#13482=ORIENTED_EDGE('',*,*,#9842,.F.);
#13483=ORIENTED_EDGE('',*,*,#9844,.F.);
#13484=ORIENTED_EDGE('',*,*,#9845,.T.);
#13485=ORIENTED_EDGE('',*,*,#9723,.F.);
#13486=ORIENTED_EDGE('',*,*,#9846,.F.);
#13487=ORIENTED_EDGE('',*,*,#9756,.T.);
#13488=ORIENTED_EDGE('',*,*,#9847,.T.);
#13489=ORIENTED_EDGE('',*,*,#9848,.F.);
#13490=ORIENTED_EDGE('',*,*,#9727,.T.);
#13491=ORIENTED_EDGE('',*,*,#9762,.T.);
#13492=ORIENTED_EDGE('',*,*,#9763,.T.);
#13493=ORIENTED_EDGE('',*,*,#9849,.T.);
#13494=ORIENTED_EDGE('',*,*,#9845,.F.);
#13495=ORIENTED_EDGE('',*,*,#9850,.F.);
#13496=ORIENTED_EDGE('',*,*,#9851,.T.);
#13497=ORIENTED_EDGE('',*,*,#9852,.T.);
#13498=ORIENTED_EDGE('',*,*,#9724,.F.);
#13499=ORIENTED_EDGE('',*,*,#9851,.F.);
#13500=ORIENTED_EDGE('',*,*,#9853,.F.);
#13501=ORIENTED_EDGE('',*,*,#9854,.T.);
#13502=ORIENTED_EDGE('',*,*,#9725,.F.);
#13503=ORIENTED_EDGE('',*,*,#9852,.F.);
#13504=ORIENTED_EDGE('',*,*,#9855,.F.);
#13505=ORIENTED_EDGE('',*,*,#9856,.T.);
#13506=ORIENTED_EDGE('',*,*,#9857,.F.);
#13507=ORIENTED_EDGE('',*,*,#9767,.T.);
#13508=ORIENTED_EDGE('',*,*,#9752,.T.);
#13509=ORIENTED_EDGE('',*,*,#9730,.T.);
#13510=ORIENTED_EDGE('',*,*,#9748,.T.);
#13511=ORIENTED_EDGE('',*,*,#9858,.F.);
#13512=ORIENTED_EDGE('',*,*,#9859,.F.);
#13513=ORIENTED_EDGE('',*,*,#9860,.T.);
#13514=ORIENTED_EDGE('',*,*,#9856,.F.);
#13515=ORIENTED_EDGE('',*,*,#9861,.F.);
#13516=ORIENTED_EDGE('',*,*,#9862,.T.);
#13517=ORIENTED_EDGE('',*,*,#9863,.T.);
#13518=ORIENTED_EDGE('',*,*,#9862,.F.);
#13519=ORIENTED_EDGE('',*,*,#9864,.F.);
#13520=ORIENTED_EDGE('',*,*,#9865,.T.);
#13521=ORIENTED_EDGE('',*,*,#9858,.T.);
#13522=ORIENTED_EDGE('',*,*,#9750,.T.);
#13523=ORIENTED_EDGE('',*,*,#9866,.T.);
#13524=ORIENTED_EDGE('',*,*,#9865,.F.);
#13525=ORIENTED_EDGE('',*,*,#9867,.F.);
#13526=ORIENTED_EDGE('',*,*,#9868,.F.);
#13527=ORIENTED_EDGE('',*,*,#9757,.T.);
#13528=ORIENTED_EDGE('',*,*,#9846,.T.);
#13529=ORIENTED_EDGE('',*,*,#9722,.F.);
#13530=ORIENTED_EDGE('',*,*,#9854,.F.);
#13531=ORIENTED_EDGE('',*,*,#9869,.T.);
#13532=ORIENTED_EDGE('',*,*,#9847,.F.);
#13533=ORIENTED_EDGE('',*,*,#9755,.T.);
#13534=ORIENTED_EDGE('',*,*,#9870,.F.);
#13535=ORIENTED_EDGE('',*,*,#9815,.T.);
#13536=ORIENTED_EDGE('',*,*,#9848,.T.);
#13537=ORIENTED_EDGE('',*,*,#9869,.F.);
#13538=ORIENTED_EDGE('',*,*,#9814,.F.);
#13539=ORIENTED_EDGE('',*,*,#9818,.F.);
#13540=ORIENTED_EDGE('',*,*,#9822,.F.);
#13541=ORIENTED_EDGE('',*,*,#9664,.T.);
#13542=ORIENTED_EDGE('',*,*,#9823,.F.);
#13543=ORIENTED_EDGE('',*,*,#9826,.F.);
#13544=ORIENTED_EDGE('',*,*,#9830,.F.);
#13545=ORIENTED_EDGE('',*,*,#9668,.T.);
#13546=ORIENTED_EDGE('',*,*,#9831,.F.);
#13547=ORIENTED_EDGE('',*,*,#9834,.F.);
#13548=ORIENTED_EDGE('',*,*,#9837,.F.);
#13549=ORIENTED_EDGE('',*,*,#9840,.F.);
#13550=ORIENTED_EDGE('',*,*,#9843,.F.);
#13551=ORIENTED_EDGE('',*,*,#9849,.F.);
#13552=ORIENTED_EDGE('',*,*,#9768,.T.);
#13553=ORIENTED_EDGE('',*,*,#9857,.T.);
#13554=ORIENTED_EDGE('',*,*,#9860,.F.);
#13555=ORIENTED_EDGE('',*,*,#9863,.F.);
#13556=ORIENTED_EDGE('',*,*,#9866,.F.);
#13557=ORIENTED_EDGE('',*,*,#9749,.T.);
#13558=ORIENTED_EDGE('',*,*,#9728,.T.);
#13559=ORIENTED_EDGE('',*,*,#9811,.T.);
#13560=ORIENTED_EDGE('',*,*,#9771,.T.);
#13561=ORIENTED_EDGE('',*,*,#9648,.T.);
#13562=ORIENTED_EDGE('',*,*,#9778,.T.);
#13563=ORIENTED_EDGE('',*,*,#9652,.T.);
#13564=ORIENTED_EDGE('',*,*,#9776,.T.);
#13565=ORIENTED_EDGE('',*,*,#9656,.T.);
#13566=ORIENTED_EDGE('',*,*,#9774,.T.);
#13567=ORIENTED_EDGE('',*,*,#9660,.T.);
#13568=ORIENTED_EDGE('',*,*,#9813,.T.);
#13569=ORIENTED_EDGE('',*,*,#9809,.T.);
#13570=ORIENTED_EDGE('',*,*,#9807,.T.);
#13571=ORIENTED_EDGE('',*,*,#9805,.T.);
#13572=ORIENTED_EDGE('',*,*,#9803,.T.);
#13573=ORIENTED_EDGE('',*,*,#9801,.T.);
#13574=ORIENTED_EDGE('',*,*,#9799,.T.);
#13575=ORIENTED_EDGE('',*,*,#9797,.T.);
#13576=ORIENTED_EDGE('',*,*,#9795,.T.);
#13577=ORIENTED_EDGE('',*,*,#9792,.T.);
#13578=ORIENTED_EDGE('',*,*,#9789,.T.);
#13579=ORIENTED_EDGE('',*,*,#9787,.T.);
#13580=ORIENTED_EDGE('',*,*,#9785,.T.);
#13581=ORIENTED_EDGE('',*,*,#9783,.T.);
#13582=ORIENTED_EDGE('',*,*,#9780,.T.);
#13583=ORIENTED_EDGE('',*,*,#9870,.T.);
#13584=ORIENTED_EDGE('',*,*,#9758,.T.);
#13585=ORIENTED_EDGE('',*,*,#9868,.T.);
#13586=ORIENTED_EDGE('',*,*,#9859,.T.);
#13587=ORIENTED_EDGE('',*,*,#9867,.T.);
#13588=ORIENTED_EDGE('',*,*,#9864,.T.);
#13589=ORIENTED_EDGE('',*,*,#9861,.T.);
#13590=ORIENTED_EDGE('',*,*,#9855,.T.);
#13591=ORIENTED_EDGE('',*,*,#9853,.T.);
#13592=ORIENTED_EDGE('',*,*,#9850,.T.);
#13593=ORIENTED_EDGE('',*,*,#9844,.T.);
#13594=ORIENTED_EDGE('',*,*,#9841,.T.);
#13595=ORIENTED_EDGE('',*,*,#9838,.T.);
#13596=ORIENTED_EDGE('',*,*,#9835,.T.);
#13597=ORIENTED_EDGE('',*,*,#9832,.T.);
#13598=ORIENTED_EDGE('',*,*,#9666,.T.);
#13599=ORIENTED_EDGE('',*,*,#9829,.T.);
#13600=ORIENTED_EDGE('',*,*,#9827,.T.);
#13601=ORIENTED_EDGE('',*,*,#9824,.T.);
#13602=ORIENTED_EDGE('',*,*,#9662,.T.);
#13603=ORIENTED_EDGE('',*,*,#9821,.T.);
#13604=ORIENTED_EDGE('',*,*,#9819,.T.);
#13605=ORIENTED_EDGE('',*,*,#9816,.T.);
#13606=ORIENTED_EDGE('',*,*,#9775,.F.);
#13607=ORIENTED_EDGE('',*,*,#9650,.T.);
#13608=ORIENTED_EDGE('',*,*,#9777,.F.);
#13609=ORIENTED_EDGE('',*,*,#9646,.T.);
#13610=ORIENTED_EDGE('',*,*,#9772,.F.);
#13611=ORIENTED_EDGE('',*,*,#9658,.T.);
#13612=ORIENTED_EDGE('',*,*,#9773,.F.);
#13613=ORIENTED_EDGE('',*,*,#9654,.T.);
#13614=ORIENTED_EDGE('',*,*,#9793,.F.);
#13615=ORIENTED_EDGE('',*,*,#9790,.F.);
#13616=ORIENTED_EDGE('',*,*,#9781,.F.);
#13617=ORIENTED_EDGE('',*,*,#9673,.T.);
#13618=ORIENTED_EDGE('',*,*,#9677,.T.);
#13619=ORIENTED_EDGE('',*,*,#9681,.T.);
#13620=ORIENTED_EDGE('',*,*,#9685,.T.);
#13621=ORIENTED_EDGE('',*,*,#9689,.T.);
#13622=ORIENTED_EDGE('',*,*,#9693,.T.);
#13623=ORIENTED_EDGE('',*,*,#9697,.T.);
#13624=ORIENTED_EDGE('',*,*,#9701,.T.);
#13625=ORIENTED_EDGE('',*,*,#9705,.T.);
#13626=ORIENTED_EDGE('',*,*,#9709,.T.);
#13627=ORIENTED_EDGE('',*,*,#9713,.T.);
#13628=ORIENTED_EDGE('',*,*,#9717,.T.);
#13629=ORIENTED_EDGE('',*,*,#9721,.T.);
#13630=ORIENTED_EDGE('',*,*,#9732,.F.);
#13631=ORIENTED_EDGE('',*,*,#9751,.T.);
#13632=ORIENTED_EDGE('',*,*,#9747,.T.);
#13633=ORIENTED_EDGE('',*,*,#9871,.T.);
#13634=ORIENTED_EDGE('',*,*,#9733,.F.);
#13635=ORIENTED_EDGE('',*,*,#9871,.F.);
#13636=ORIENTED_EDGE('',*,*,#9746,.T.);
#13637=ORIENTED_EDGE('',*,*,#9872,.T.);
#13638=ORIENTED_EDGE('',*,*,#9734,.F.);
#13639=ORIENTED_EDGE('',*,*,#9872,.F.);
#13640=ORIENTED_EDGE('',*,*,#9745,.F.);
#13641=ORIENTED_EDGE('',*,*,#9759,.T.);
#16520=PLANE('',#18635);
#16521=PLANE('',#18636);
#16522=PLANE('',#18640);
#16523=PLANE('',#18641);
#16524=PLANE('',#18642);
#16525=PLANE('',#18643);
#16526=PLANE('',#18653);
#16527=PLANE('',#18654);
#16528=PLANE('',#18655);
#16529=PLANE('',#18656);
#16530=PLANE('',#18657);
#16531=PLANE('',#18658);
#16532=PLANE('',#18659);
#16533=PLANE('',#18660);
#16534=PLANE('',#18696);
#16535=PLANE('',#18697);
#16536=PLANE('',#18698);
#16537=PLANE('',#18699);
#16538=PLANE('',#18703);
#16539=PLANE('',#18704);
#16540=PLANE('',#18708);
#16541=PLANE('',#18712);
#16542=PLANE('',#18713);
#16543=PLANE('',#18714);
#16544=PLANE('',#18715);
#16545=PLANE('',#18716);
#16546=PLANE('',#18717);
#16547=PLANE('',#18718);
#16548=PLANE('',#18719);
#16549=PLANE('',#18720);
#16550=PLANE('',#18721);
#16551=PLANE('',#18722);
#16552=PLANE('',#18723);
#16553=PLANE('',#18724);
#16554=PLANE('',#18725);
#17215=ADVANCED_FACE('',(#1880),#585,.F.);
#17216=ADVANCED_FACE('',(#1881),#586,.F.);
#17217=ADVANCED_FACE('',(#1882),#587,.F.);
#17218=ADVANCED_FACE('',(#1883),#588,.F.);
#17219=ADVANCED_FACE('',(#1884),#589,.F.);
#17220=ADVANCED_FACE('',(#1885),#590,.F.);
#17221=ADVANCED_FACE('',(#1886),#171,.F.);
#17222=ADVANCED_FACE('',(#1887),#172,.F.);
#17223=ADVANCED_FACE('',(#1888),#173,.F.);
#17224=ADVANCED_FACE('',(#1889),#174,.F.);
#17225=ADVANCED_FACE('',(#1890),#175,.F.);
#17226=ADVANCED_FACE('',(#1891),#176,.F.);
#17227=ADVANCED_FACE('',(#1892),#177,.F.);
#17228=ADVANCED_FACE('',(#1893),#178,.F.);
#17229=ADVANCED_FACE('',(#1894),#179,.F.);
#17230=ADVANCED_FACE('',(#1895),#180,.F.);
#17231=ADVANCED_FACE('',(#1896),#181,.F.);
#17232=ADVANCED_FACE('',(#1897),#182,.F.);
#17233=ADVANCED_FACE('',(#1898),#183,.F.);
#17234=ADVANCED_FACE('',(#1899),#16520,.F.);
#17235=ADVANCED_FACE('',(#1900),#16521,.F.);
#17236=ADVANCED_FACE('',(#1901),#16522,.F.);
#17237=ADVANCED_FACE('',(#1902),#16523,.F.);
#17238=ADVANCED_FACE('',(#1903),#16524,.F.);
#17239=ADVANCED_FACE('',(#1904),#16525,.F.);
#17240=ADVANCED_FACE('',(#1905),#591,.F.);
#17241=ADVANCED_FACE('',(#1906),#592,.F.);
#17242=ADVANCED_FACE('',(#1907),#593,.T.);
#17243=ADVANCED_FACE('',(#1908),#594,.T.);
#17244=ADVANCED_FACE('',(#1909),#16526,.T.);
#17245=ADVANCED_FACE('',(#1910),#16527,.T.);
#17246=ADVANCED_FACE('',(#1911),#16528,.T.);
#17247=ADVANCED_FACE('',(#1912),#16529,.T.);
#17248=ADVANCED_FACE('',(#1913),#16530,.T.);
#17249=ADVANCED_FACE('',(#1914),#16531,.T.);
#17250=ADVANCED_FACE('',(#1915),#16532,.T.);
#17251=ADVANCED_FACE('',(#1916),#16533,.T.);
#17252=ADVANCED_FACE('',(#1917),#595,.F.);
#17253=ADVANCED_FACE('',(#1918),#596,.F.);
#17254=ADVANCED_FACE('',(#1919),#597,.F.);
#17255=ADVANCED_FACE('',(#1920),#598,.F.);
#17256=ADVANCED_FACE('',(#1921),#599,.F.);
#17257=ADVANCED_FACE('',(#1922),#600,.F.);
#17258=ADVANCED_FACE('',(#1923),#601,.F.);
#17259=ADVANCED_FACE('',(#1924),#602,.F.);
#17260=ADVANCED_FACE('',(#1925),#603,.F.);
#17261=ADVANCED_FACE('',(#1926),#604,.F.);
#17262=ADVANCED_FACE('',(#1927),#605,.F.);
#17263=ADVANCED_FACE('',(#1928),#606,.F.);
#17264=ADVANCED_FACE('',(#1929),#607,.F.);
#17265=ADVANCED_FACE('',(#1930),#608,.F.);
#17266=ADVANCED_FACE('',(#1931),#609,.F.);
#17267=ADVANCED_FACE('',(#1932),#610,.F.);
#17268=ADVANCED_FACE('',(#1933),#16534,.F.);
#17269=ADVANCED_FACE('',(#1934),#16535,.F.);
#17270=ADVANCED_FACE('',(#1935),#16536,.F.);
#17271=ADVANCED_FACE('',(#1936),#16537,.F.);
#17272=ADVANCED_FACE('',(#1937),#611,.T.);
#17273=ADVANCED_FACE('',(#1938),#16538,.F.);
#17274=ADVANCED_FACE('',(#1939),#16539,.F.);
#17275=ADVANCED_FACE('',(#1940),#612,.T.);
#17276=ADVANCED_FACE('',(#1941),#16540,.F.);
#17277=ADVANCED_FACE('',(#1942),#613,.T.);
#17278=ADVANCED_FACE('',(#1943),#16541,.F.);
#17279=ADVANCED_FACE('',(#1944),#16542,.F.);
#17280=ADVANCED_FACE('',(#1945),#16543,.F.);
#17281=ADVANCED_FACE('',(#1946),#16544,.F.);
#17282=ADVANCED_FACE('',(#1947),#16545,.F.);
#17283=ADVANCED_FACE('',(#1948),#16546,.F.);
#17284=ADVANCED_FACE('',(#1949),#16547,.F.);
#17285=ADVANCED_FACE('',(#1950),#16548,.F.);
#17286=ADVANCED_FACE('',(#1951),#16549,.F.);
#17287=ADVANCED_FACE('',(#1952,#891,#892,#893,#894,#895,#896,#897,#898,
#899,#900,#901,#902,#903,#904,#905,#906,#907),#16550,.F.);
#17288=ADVANCED_FACE('',(#1953,#908,#909,#910,#911,#912,#913,#914,#915,
#916,#917,#918,#919,#920,#921,#922,#923,#924),#16551,.T.);
#17289=ADVANCED_FACE('',(#1954),#16552,.T.);
#17290=ADVANCED_FACE('',(#1955),#16553,.T.);
#17291=ADVANCED_FACE('',(#1956),#16554,.T.);
#17796=CLOSED_SHELL('',(#17215,#17216,#17217,#17218,#17219,#17220,#17221,
#17222,#17223,#17224,#17225,#17226,#17227,#17228,#17229,#17230,#17231,#17232,
#17233,#17234,#17235,#17236,#17237,#17238,#17239,#17240,#17241,#17242,#17243,
#17244,#17245,#17246,#17247,#17248,#17249,#17250,#17251,#17252,#17253,#17254,
#17255,#17256,#17257,#17258,#17259,#17260,#17261,#17262,#17263,#17264,#17265,
#17266,#17267,#17268,#17269,#17270,#17271,#17272,#17273,#17274,#17275,#17276,
#17277,#17278,#17279,#17280,#17281,#17282,#17283,#17284,#17285,#17286,#17287,
#17288,#17289,#17290,#17291));
#18564=AXIS2_PLACEMENT_3D('',#26841,#21379,#21380);
#18565=AXIS2_PLACEMENT_3D('',#26842,#21381,#21382);
#18566=AXIS2_PLACEMENT_3D('',#26845,#21383,#21384);
#18567=AXIS2_PLACEMENT_3D('',#26849,#21386,#21387);
#18568=AXIS2_PLACEMENT_3D('',#26851,#21389,#21390);
#18569=AXIS2_PLACEMENT_3D('',#26854,#21391,#21392);
#18570=AXIS2_PLACEMENT_3D('',#26858,#21394,#21395);
#18571=AXIS2_PLACEMENT_3D('',#26860,#21397,#21398);
#18572=AXIS2_PLACEMENT_3D('',#26863,#21399,#21400);
#18573=AXIS2_PLACEMENT_3D('',#26867,#21402,#21403);
#18574=AXIS2_PLACEMENT_3D('',#26869,#21405,#21406);
#18575=AXIS2_PLACEMENT_3D('',#26872,#21407,#21408);
#18576=AXIS2_PLACEMENT_3D('',#26876,#21410,#21411);
#18577=AXIS2_PLACEMENT_3D('',#26878,#21413,#21414);
#18578=AXIS2_PLACEMENT_3D('',#26881,#21415,#21416);
#18579=AXIS2_PLACEMENT_3D('',#26885,#21418,#21419);
#18580=AXIS2_PLACEMENT_3D('',#26887,#21421,#21422);
#18581=AXIS2_PLACEMENT_3D('',#26890,#21423,#21424);
#18582=AXIS2_PLACEMENT_3D('',#26894,#21426,#21427);
#18583=AXIS2_PLACEMENT_3D('',#26896,#21429,#21430);
#18584=AXIS2_PLACEMENT_3D('',#26899,#21431,#21432);
#18585=AXIS2_PLACEMENT_3D('',#26900,#21433,#21434);
#18586=AXIS2_PLACEMENT_3D('',#26903,#21436,#21437);
#18587=AXIS2_PLACEMENT_3D('',#26904,#21438,#21439);
#18588=AXIS2_PLACEMENT_3D('',#26907,#21440,#21441);
#18589=AXIS2_PLACEMENT_3D('',#26908,#21442,#21443);
#18590=AXIS2_PLACEMENT_3D('',#26911,#21445,#21446);
#18591=AXIS2_PLACEMENT_3D('',#26912,#21447,#21448);
#18592=AXIS2_PLACEMENT_3D('',#26915,#21449,#21450);
#18593=AXIS2_PLACEMENT_3D('',#26916,#21451,#21452);
#18594=AXIS2_PLACEMENT_3D('',#26919,#21454,#21455);
#18595=AXIS2_PLACEMENT_3D('',#26920,#21456,#21457);
#18596=AXIS2_PLACEMENT_3D('',#26923,#21458,#21459);
#18597=AXIS2_PLACEMENT_3D('',#26924,#21460,#21461);
#18598=AXIS2_PLACEMENT_3D('',#26927,#21463,#21464);
#18599=AXIS2_PLACEMENT_3D('',#26928,#21465,#21466);
#18600=AXIS2_PLACEMENT_3D('',#26931,#21467,#21468);
#18601=AXIS2_PLACEMENT_3D('',#26932,#21469,#21470);
#18602=AXIS2_PLACEMENT_3D('',#26935,#21472,#21473);
#18603=AXIS2_PLACEMENT_3D('',#26936,#21474,#21475);
#18604=AXIS2_PLACEMENT_3D('',#26939,#21476,#21477);
#18605=AXIS2_PLACEMENT_3D('',#26940,#21478,#21479);
#18606=AXIS2_PLACEMENT_3D('',#26943,#21481,#21482);
#18607=AXIS2_PLACEMENT_3D('',#26944,#21483,#21484);
#18608=AXIS2_PLACEMENT_3D('',#26947,#21485,#21486);
#18609=AXIS2_PLACEMENT_3D('',#26948,#21487,#21488);
#18610=AXIS2_PLACEMENT_3D('',#26951,#21490,#21491);
#18611=AXIS2_PLACEMENT_3D('',#26952,#21492,#21493);
#18612=AXIS2_PLACEMENT_3D('',#26955,#21494,#21495);
#18613=AXIS2_PLACEMENT_3D('',#26956,#21496,#21497);
#18614=AXIS2_PLACEMENT_3D('',#26959,#21499,#21500);
#18615=AXIS2_PLACEMENT_3D('',#26960,#21501,#21502);
#18616=AXIS2_PLACEMENT_3D('',#26963,#21503,#21504);
#18617=AXIS2_PLACEMENT_3D('',#26964,#21505,#21506);
#18618=AXIS2_PLACEMENT_3D('',#26967,#21508,#21509);
#18619=AXIS2_PLACEMENT_3D('',#26968,#21510,#21511);
#18620=AXIS2_PLACEMENT_3D('',#26971,#21512,#21513);
#18621=AXIS2_PLACEMENT_3D('',#26972,#21514,#21515);
#18622=AXIS2_PLACEMENT_3D('',#26975,#21517,#21518);
#18623=AXIS2_PLACEMENT_3D('',#26976,#21519,#21520);
#18624=AXIS2_PLACEMENT_3D('',#26979,#21521,#21522);
#18625=AXIS2_PLACEMENT_3D('',#26980,#21523,#21524);
#18626=AXIS2_PLACEMENT_3D('',#26983,#21526,#21527);
#18627=AXIS2_PLACEMENT_3D('',#26984,#21528,#21529);
#18628=AXIS2_PLACEMENT_3D('',#26987,#21530,#21531);
#18629=AXIS2_PLACEMENT_3D('',#26988,#21532,#21533);
#18630=AXIS2_PLACEMENT_3D('',#26991,#21535,#21536);
#18631=AXIS2_PLACEMENT_3D('',#26992,#21537,#21538);
#18632=AXIS2_PLACEMENT_3D('',#26995,#21539,#21540);
#18633=AXIS2_PLACEMENT_3D('',#26996,#21541,#21542);
#18634=AXIS2_PLACEMENT_3D('',#26999,#21544,#21545);
#18635=AXIS2_PLACEMENT_3D('',#27000,#21546,#21547);
#18636=AXIS2_PLACEMENT_3D('',#27009,#21552,#21553);
#18637=AXIS2_PLACEMENT_3D('',#27012,#21554,#21555);
#18638=AXIS2_PLACEMENT_3D('',#27018,#21558,#21559);
#18639=AXIS2_PLACEMENT_3D('',#27022,#21561,#21562);
#18640=AXIS2_PLACEMENT_3D('',#27028,#21566,#21567);
#18641=AXIS2_PLACEMENT_3D('',#27037,#21572,#21573);
#18642=AXIS2_PLACEMENT_3D('',#27045,#21578,#21579);
#18643=AXIS2_PLACEMENT_3D('',#27049,#21582,#21583);
#18644=AXIS2_PLACEMENT_3D('',#27055,#21587,#21588);
#18645=AXIS2_PLACEMENT_3D('',#27060,#21591,#21592);
#18646=AXIS2_PLACEMENT_3D('',#27061,#21593,#21594);
#18647=AXIS2_PLACEMENT_3D('',#27066,#21597,#21598);
#18648=AXIS2_PLACEMENT_3D('',#27068,#21600,#21601);
#18649=AXIS2_PLACEMENT_3D('',#27071,#21602,#21603);
#18650=AXIS2_PLACEMENT_3D('',#27075,#21605,#21606);
#18651=AXIS2_PLACEMENT_3D('',#27077,#21608,#21609);
#18652=AXIS2_PLACEMENT_3D('',#27082,#21612,#21613);
#18653=AXIS2_PLACEMENT_3D('',#27084,#21615,#21616);
#18654=AXIS2_PLACEMENT_3D('',#27095,#21623,#21624);
#18655=AXIS2_PLACEMENT_3D('',#27097,#21626,#21627);
#18656=AXIS2_PLACEMENT_3D('',#27099,#21629,#21630);
#18657=AXIS2_PLACEMENT_3D('',#27100,#21631,#21632);
#18658=AXIS2_PLACEMENT_3D('',#27103,#21635,#21636);
#18659=AXIS2_PLACEMENT_3D('',#27106,#21639,#21640);
#18660=AXIS2_PLACEMENT_3D('',#27109,#21643,#21644);
#18661=AXIS2_PLACEMENT_3D('',#27112,#21647,#21648);
#18662=AXIS2_PLACEMENT_3D('',#27115,#21650,#21651);
#18663=AXIS2_PLACEMENT_3D('',#27116,#21652,#21653);
#18664=AXIS2_PLACEMENT_3D('',#27118,#21654,#21655);
#18665=AXIS2_PLACEMENT_3D('',#27121,#21657,#21658);
#18666=AXIS2_PLACEMENT_3D('',#27122,#21659,#21660);
#18667=AXIS2_PLACEMENT_3D('',#27125,#21662,#21663);
#18668=AXIS2_PLACEMENT_3D('',#27126,#21664,#21665);
#18669=AXIS2_PLACEMENT_3D('',#27129,#21667,#21668);
#18670=AXIS2_PLACEMENT_3D('',#27130,#21669,#21670);
#18671=AXIS2_PLACEMENT_3D('',#27133,#21672,#21673);
#18672=AXIS2_PLACEMENT_3D('',#27134,#21674,#21675);
#18673=AXIS2_PLACEMENT_3D('',#27136,#21676,#21677);
#18674=AXIS2_PLACEMENT_3D('',#27139,#21679,#21680);
#18675=AXIS2_PLACEMENT_3D('',#27140,#21681,#21682);
#18676=AXIS2_PLACEMENT_3D('',#27142,#21683,#21684);
#18677=AXIS2_PLACEMENT_3D('',#27145,#21686,#21687);
#18678=AXIS2_PLACEMENT_3D('',#27146,#21688,#21689);
#18679=AXIS2_PLACEMENT_3D('',#27149,#21691,#21692);
#18680=AXIS2_PLACEMENT_3D('',#27150,#21693,#21694);
#18681=AXIS2_PLACEMENT_3D('',#27153,#21696,#21697);
#18682=AXIS2_PLACEMENT_3D('',#27154,#21698,#21699);
#18683=AXIS2_PLACEMENT_3D('',#27157,#21701,#21702);
#18684=AXIS2_PLACEMENT_3D('',#27158,#21703,#21704);
#18685=AXIS2_PLACEMENT_3D('',#27161,#21706,#21707);
#18686=AXIS2_PLACEMENT_3D('',#27162,#21708,#21709);
#18687=AXIS2_PLACEMENT_3D('',#27165,#21711,#21712);
#18688=AXIS2_PLACEMENT_3D('',#27166,#21713,#21714);
#18689=AXIS2_PLACEMENT_3D('',#27169,#21716,#21717);
#18690=AXIS2_PLACEMENT_3D('',#27170,#21718,#21719);
#18691=AXIS2_PLACEMENT_3D('',#27173,#21721,#21722);
#18692=AXIS2_PLACEMENT_3D('',#27174,#21723,#21724);
#18693=AXIS2_PLACEMENT_3D('',#27177,#21726,#21727);
#18694=AXIS2_PLACEMENT_3D('',#27178,#21728,#21729);
#18695=AXIS2_PLACEMENT_3D('',#27181,#21731,#21732);
#18696=AXIS2_PLACEMENT_3D('',#27182,#21733,#21734);
#18697=AXIS2_PLACEMENT_3D('',#27191,#21739,#21740);
#18698=AXIS2_PLACEMENT_3D('',#27197,#21744,#21745);
#18699=AXIS2_PLACEMENT_3D('',#27200,#21748,#21749);
#18700=AXIS2_PLACEMENT_3D('',#27206,#21753,#21754);
#18701=AXIS2_PLACEMENT_3D('',#27208,#21755,#21756);
#18702=AXIS2_PLACEMENT_3D('',#27210,#21757,#21758);
#18703=AXIS2_PLACEMENT_3D('',#27212,#21760,#21761);
#18704=AXIS2_PLACEMENT_3D('',#27215,#21764,#21765);
#18705=AXIS2_PLACEMENT_3D('',#27221,#21769,#21770);
#18706=AXIS2_PLACEMENT_3D('',#27223,#21771,#21772);
#18707=AXIS2_PLACEMENT_3D('',#27225,#21773,#21774);
#18708=AXIS2_PLACEMENT_3D('',#27227,#21776,#21777);
#18709=AXIS2_PLACEMENT_3D('',#27233,#21781,#21782);
#18710=AXIS2_PLACEMENT_3D('',#27235,#21783,#21784);
#18711=AXIS2_PLACEMENT_3D('',#27237,#21785,#21786);
#18712=AXIS2_PLACEMENT_3D('',#27239,#21788,#21789);
#18713=AXIS2_PLACEMENT_3D('',#27245,#21793,#21794);
#18714=AXIS2_PLACEMENT_3D('',#27254,#21801,#21802);
#18715=AXIS2_PLACEMENT_3D('',#27258,#21805,#21806);
#18716=AXIS2_PLACEMENT_3D('',#27269,#21813,#21814);
#18717=AXIS2_PLACEMENT_3D('',#27275,#21818,#21819);
#18718=AXIS2_PLACEMENT_3D('',#27281,#21823,#21824);
#18719=AXIS2_PLACEMENT_3D('',#27284,#21827,#21828);
#18720=AXIS2_PLACEMENT_3D('',#27286,#21830,#21831);
#18721=AXIS2_PLACEMENT_3D('',#27289,#21834,#21835);
#18722=AXIS2_PLACEMENT_3D('',#27290,#21836,#21837);
#18723=AXIS2_PLACEMENT_3D('',#27291,#21838,#21839);
#18724=AXIS2_PLACEMENT_3D('',#27293,#21841,#21842);
#18725=AXIS2_PLACEMENT_3D('',#27295,#21844,#21845);
#21379=DIRECTION('axis',(0.,0.,1.));
#21380=DIRECTION('refdir',(1.,0.,0.));
#21381=DIRECTION('center_axis',(0.,0.,1.));
#21382=DIRECTION('ref_axis',(1.,0.,0.));
#21383=DIRECTION('center_axis',(0.,0.,-1.));
#21384=DIRECTION('ref_axis',(1.,0.,0.));
#21385=DIRECTION('',(0.,0.,1.));
#21386=DIRECTION('center_axis',(0.,0.,1.));
#21387=DIRECTION('ref_axis',(1.,0.,0.));
#21388=DIRECTION('',(0.,0.,-1.));
#21389=DIRECTION('center_axis',(0.,0.,1.));
#21390=DIRECTION('ref_axis',(1.,0.,0.));
#21391=DIRECTION('center_axis',(0.,0.,-1.));
#21392=DIRECTION('ref_axis',(1.,0.,0.));
#21393=DIRECTION('',(0.,0.,1.));
#21394=DIRECTION('center_axis',(0.,0.,1.));
#21395=DIRECTION('ref_axis',(1.,0.,0.));
#21396=DIRECTION('',(0.,0.,-1.));
#21397=DIRECTION('center_axis',(0.,0.,1.));
#21398=DIRECTION('ref_axis',(1.,0.,0.));
#21399=DIRECTION('center_axis',(0.,0.,-1.));
#21400=DIRECTION('ref_axis',(1.,0.,0.));
#21401=DIRECTION('',(0.,0.,1.));
#21402=DIRECTION('center_axis',(0.,0.,1.));
#21403=DIRECTION('ref_axis',(1.,0.,0.));
#21404=DIRECTION('',(0.,0.,-1.));
#21405=DIRECTION('center_axis',(0.,0.,1.));
#21406=DIRECTION('ref_axis',(1.,0.,0.));
#21407=DIRECTION('center_axis',(0.,0.,-1.));
#21408=DIRECTION('ref_axis',(1.,0.,0.));
#21409=DIRECTION('',(0.,0.,1.));
#21410=DIRECTION('center_axis',(0.,0.,1.));
#21411=DIRECTION('ref_axis',(1.,0.,0.));
#21412=DIRECTION('',(0.,0.,-1.));
#21413=DIRECTION('center_axis',(0.,0.,1.));
#21414=DIRECTION('ref_axis',(1.,0.,0.));
#21415=DIRECTION('center_axis',(0.,0.,-1.));
#21416=DIRECTION('ref_axis',(1.,0.,0.));
#21417=DIRECTION('',(0.,0.,1.));
#21418=DIRECTION('center_axis',(0.,0.,1.));
#21419=DIRECTION('ref_axis',(1.,0.,0.));
#21420=DIRECTION('',(0.,0.,-1.));
#21421=DIRECTION('center_axis',(0.,0.,1.));
#21422=DIRECTION('ref_axis',(1.,0.,0.));
#21423=DIRECTION('center_axis',(0.,0.,-1.));
#21424=DIRECTION('ref_axis',(1.,6.93889390390722E-15,0.));
#21425=DIRECTION('',(0.,0.,1.));
#21426=DIRECTION('center_axis',(0.,0.,1.));
#21427=DIRECTION('ref_axis',(1.,0.,0.));
#21428=DIRECTION('',(0.,0.,-1.));
#21429=DIRECTION('center_axis',(0.,0.,1.));
#21430=DIRECTION('ref_axis',(1.,0.,0.));
#21431=DIRECTION('center_axis',(0.,0.,1.));
#21432=DIRECTION('ref_axis',(1.,0.,0.));
#21433=DIRECTION('center_axis',(0.,0.,1.));
#21434=DIRECTION('ref_axis',(1.,0.,0.));
#21435=DIRECTION('',(-0.707106781186554,-8.65956056235502E-17,0.707106781186541));
#21436=DIRECTION('center_axis',(0.,0.,-1.));
#21437=DIRECTION('ref_axis',(1.,0.,0.));
#21438=DIRECTION('center_axis',(0.,0.,1.));
#21439=DIRECTION('ref_axis',(1.,0.,0.));
#21440=DIRECTION('center_axis',(0.,0.,1.));
#21441=DIRECTION('ref_axis',(1.,0.,0.));
#21442=DIRECTION('center_axis',(0.,0.,1.));
#21443=DIRECTION('ref_axis',(1.,0.,0.));
#21444=DIRECTION('',(-0.707106781186554,-8.65956056235501E-17,0.707106781186541));
#21445=DIRECTION('center_axis',(0.,0.,-1.));
#21446=DIRECTION('ref_axis',(1.,0.,0.));
#21447=DIRECTION('center_axis',(0.,0.,1.));
#21448=DIRECTION('ref_axis',(1.,0.,0.));
#21449=DIRECTION('center_axis',(0.,0.,1.));
#21450=DIRECTION('ref_axis',(1.,0.,0.));
#21451=DIRECTION('center_axis',(0.,0.,1.));
#21452=DIRECTION('ref_axis',(1.,0.,0.));
#21453=DIRECTION('',(-0.707106781186554,-8.65956056235502E-17,0.707106781186541));
#21454=DIRECTION('center_axis',(0.,0.,-1.));
#21455=DIRECTION('ref_axis',(1.,0.,0.));
#21456=DIRECTION('center_axis',(0.,0.,1.));
#21457=DIRECTION('ref_axis',(1.,0.,0.));
#21458=DIRECTION('center_axis',(0.,0.,1.));
#21459=DIRECTION('ref_axis',(1.,0.,0.));
#21460=DIRECTION('center_axis',(0.,0.,1.));
#21461=DIRECTION('ref_axis',(1.,0.,0.));
#21462=DIRECTION('',(-0.707106781186554,-8.65956056235501E-17,0.707106781186541));
#21463=DIRECTION('center_axis',(0.,0.,-1.));
#21464=DIRECTION('ref_axis',(1.,0.,0.));
#21465=DIRECTION('center_axis',(0.,0.,1.));
#21466=DIRECTION('ref_axis',(1.,0.,0.));
#21467=DIRECTION('center_axis',(0.,0.,1.));
#21468=DIRECTION('ref_axis',(1.,0.,0.));
#21469=DIRECTION('center_axis',(0.,0.,1.));
#21470=DIRECTION('ref_axis',(1.,0.,0.));
#21471=DIRECTION('',(-0.707106781186554,-8.65956056235501E-17,0.707106781186541));
#21472=DIRECTION('center_axis',(0.,0.,-1.));
#21473=DIRECTION('ref_axis',(1.,0.,0.));
#21474=DIRECTION('center_axis',(0.,0.,1.));
#21475=DIRECTION('ref_axis',(1.,0.,0.));
#21476=DIRECTION('center_axis',(0.,0.,1.));
#21477=DIRECTION('ref_axis',(1.,0.,0.));
#21478=DIRECTION('center_axis',(0.,0.,1.));
#21479=DIRECTION('ref_axis',(1.,0.,0.));
#21480=DIRECTION('',(-0.707106781186554,-8.65956056235501E-17,0.707106781186541));
#21481=DIRECTION('center_axis',(0.,0.,-1.));
#21482=DIRECTION('ref_axis',(1.,0.,0.));
#21483=DIRECTION('center_axis',(0.,0.,1.));
#21484=DIRECTION('ref_axis',(1.,0.,0.));
#21485=DIRECTION('center_axis',(0.,0.,1.));
#21486=DIRECTION('ref_axis',(1.,0.,0.));
#21487=DIRECTION('center_axis',(0.,0.,1.));
#21488=DIRECTION('ref_axis',(1.,0.,0.));
#21489=DIRECTION('',(-0.707106781186554,-8.65956056235501E-17,0.707106781186541));
#21490=DIRECTION('center_axis',(0.,0.,-1.));
#21491=DIRECTION('ref_axis',(1.,0.,0.));
#21492=DIRECTION('center_axis',(0.,0.,1.));
#21493=DIRECTION('ref_axis',(1.,0.,0.));
#21494=DIRECTION('center_axis',(0.,0.,1.));
#21495=DIRECTION('ref_axis',(1.,0.,0.));
#21496=DIRECTION('center_axis',(0.,0.,1.));
#21497=DIRECTION('ref_axis',(1.,0.,0.));
#21498=DIRECTION('',(-0.707106781186554,-8.65956056235501E-17,0.707106781186541));
#21499=DIRECTION('center_axis',(0.,0.,-1.));
#21500=DIRECTION('ref_axis',(1.,0.,0.));
#21501=DIRECTION('center_axis',(0.,0.,1.));
#21502=DIRECTION('ref_axis',(1.,0.,0.));
#21503=DIRECTION('center_axis',(0.,0.,1.));
#21504=DIRECTION('ref_axis',(1.,0.,0.));
#21505=DIRECTION('center_axis',(0.,0.,1.));
#21506=DIRECTION('ref_axis',(1.,0.,0.));
#21507=DIRECTION('',(-0.707106781186554,-8.65956056235501E-17,0.707106781186541));
#21508=DIRECTION('center_axis',(0.,0.,-1.));
#21509=DIRECTION('ref_axis',(1.,0.,0.));
#21510=DIRECTION('center_axis',(0.,0.,1.));
#21511=DIRECTION('ref_axis',(1.,0.,0.));
#21512=DIRECTION('center_axis',(0.,0.,1.));
#21513=DIRECTION('ref_axis',(1.,0.,0.));
#21514=DIRECTION('center_axis',(0.,0.,1.));
#21515=DIRECTION('ref_axis',(1.,0.,0.));
#21516=DIRECTION('',(-0.707106781186554,-8.65956056235501E-17,0.707106781186541));
#21517=DIRECTION('center_axis',(0.,0.,-1.));
#21518=DIRECTION('ref_axis',(1.,0.,0.));
#21519=DIRECTION('center_axis',(0.,0.,1.));
#21520=DIRECTION('ref_axis',(1.,0.,0.));
#21521=DIRECTION('center_axis',(0.,0.,1.));
#21522=DIRECTION('ref_axis',(1.,0.,0.));
#21523=DIRECTION('center_axis',(0.,0.,1.));
#21524=DIRECTION('ref_axis',(1.,0.,0.));
#21525=DIRECTION('',(-0.707106781186554,-8.65956056235502E-17,0.707106781186541));
#21526=DIRECTION('center_axis',(0.,0.,-1.));
#21527=DIRECTION('ref_axis',(1.,0.,0.));
#21528=DIRECTION('center_axis',(0.,0.,1.));
#21529=DIRECTION('ref_axis',(1.,0.,0.));
#21530=DIRECTION('center_axis',(0.,0.,1.));
#21531=DIRECTION('ref_axis',(1.,0.,0.));
#21532=DIRECTION('center_axis',(0.,0.,1.));
#21533=DIRECTION('ref_axis',(1.,0.,0.));
#21534=DIRECTION('',(-0.707106781186554,-8.65956056235502E-17,0.707106781186541));
#21535=DIRECTION('center_axis',(0.,0.,-1.));
#21536=DIRECTION('ref_axis',(1.,0.,0.));
#21537=DIRECTION('center_axis',(0.,0.,1.));
#21538=DIRECTION('ref_axis',(1.,0.,0.));
#21539=DIRECTION('center_axis',(0.,0.,1.));
#21540=DIRECTION('ref_axis',(1.,0.,0.));
#21541=DIRECTION('center_axis',(0.,0.,1.));
#21542=DIRECTION('ref_axis',(1.,0.,0.));
#21543=DIRECTION('',(-0.707106781186554,-8.65956056235501E-17,0.707106781186541));
#21544=DIRECTION('center_axis',(0.,0.,-1.));
#21545=DIRECTION('ref_axis',(1.,0.,0.));
#21546=DIRECTION('center_axis',(0.,0.,-1.));
#21547=DIRECTION('ref_axis',(0.,-1.,0.));
#21548=DIRECTION('',(0.,-1.,0.));
#21549=DIRECTION('',(1.,0.,0.));
#21550=DIRECTION('',(0.,1.,0.));
#21551=DIRECTION('',(-1.,0.,0.));
#21552=DIRECTION('center_axis',(1.,-4.08170229641602E-16,8.32946623846081E-32));
#21553=DIRECTION('ref_axis',(-4.08170229641602E-16,-1.,-4.19642196872632E-64));
#21554=DIRECTION('center_axis',(-1.,0.,-8.32946623846081E-32));
#21555=DIRECTION('ref_axis',(0.,1.,0.));
#21556=DIRECTION('',(-6.80579823082152E-36,-2.04085114820801E-16,-1.));
#21557=DIRECTION('',(-4.08170229641602E-16,-1.,0.));
#21558=DIRECTION('center_axis',(-1.,0.,-8.32946623846081E-32));
#21559=DIRECTION('ref_axis',(0.,1.,0.));
#21560=DIRECTION('',(-8.32946623846081E-32,-2.57814143119491E-47,1.));
#21561=DIRECTION('center_axis',(-1.,0.,-8.32946623846081E-32));
#21562=DIRECTION('ref_axis',(0.,1.,0.));
#21563=DIRECTION('',(4.08170229641602E-16,1.,-2.31296463463574E-16));
#21564=DIRECTION('',(-6.80579823082152E-36,-2.04085114820801E-16,-1.));
#21565=DIRECTION('',(-4.08170229641602E-16,-1.,2.04085114820801E-16));
#21566=DIRECTION('center_axis',(0.,2.14163392095902E-16,1.));
#21567=DIRECTION('ref_axis',(0.,-1.,2.14163392095902E-16));
#21568=DIRECTION('',(1.,3.0952060520883E-16,-7.15987345919025E-32));
#21569=DIRECTION('',(0.,-1.,2.14163392095902E-16));
#21570=DIRECTION('',(-1.,1.19262238973406E-16,0.));
#21571=DIRECTION('',(0.,1.,-2.14163392095902E-16));
#21572=DIRECTION('center_axis',(1.,-7.28776417516513E-52,-3.40289911541076E-36));
#21573=DIRECTION('ref_axis',(-3.40289911541076E-36,0.,-1.));
#21574=DIRECTION('',(0.,-1.,2.14163392095902E-16));
#21575=DIRECTION('',(-3.40289911541076E-36,-1.020425574104E-16,-1.));
#21576=DIRECTION('',(0.,-1.,2.14163392095902E-16));
#21577=DIRECTION('',(-3.40289911541076E-36,-1.020425574104E-16,-1.));
#21578=DIRECTION('center_axis',(-1.19262238973406E-16,-1.,1.020425574104E-16));
#21579=DIRECTION('ref_axis',(-1.,1.19262238973406E-16,0.));
#21580=DIRECTION('',(-1.,1.19262238973406E-16,0.));
#21581=DIRECTION('',(-3.40289911541076E-36,-1.020425574104E-16,-1.));
#21582=DIRECTION('center_axis',(-1.,7.28776417516513E-52,3.40289911541076E-36));
#21583=DIRECTION('ref_axis',(7.28776417516513E-52,1.,1.38699460815421E-104));
#21584=DIRECTION('',(0.,1.,-2.14163392095902E-16));
#21585=DIRECTION('',(-3.40289911541076E-36,-1.020425574104E-16,-1.));
#21586=DIRECTION('',(0.,1.,-2.14163392095902E-16));
#21587=DIRECTION('center_axis',(1.,0.,0.));
#21588=DIRECTION('ref_axis',(0.,1.,0.));
#21589=DIRECTION('',(1.,3.0952060520883E-16,0.));
#21590=DIRECTION('',(-1.,-3.0952060520883E-16,0.));
#21591=DIRECTION('center_axis',(-1.,0.,0.));
#21592=DIRECTION('ref_axis',(0.,-1.,0.));
#21593=DIRECTION('center_axis',(-1.,0.,7.15987345919025E-32));
#21594=DIRECTION('ref_axis',(0.,-1.,0.));
#21595=DIRECTION('',(1.,3.0952060520883E-16,-7.15987345919025E-32));
#21596=DIRECTION('',(-1.,-3.0952060520883E-16,7.15987345919025E-32));
#21597=DIRECTION('center_axis',(-1.,0.,0.));
#21598=DIRECTION('ref_axis',(0.,1.,0.));
#21599=DIRECTION('',(1.,3.0952060520883E-16,-7.15987345919025E-32));
#21600=DIRECTION('center_axis',(-1.,0.,0.));
#21601=DIRECTION('ref_axis',(0.,0.,1.));
#21602=DIRECTION('center_axis',(-1.,7.46735853138638E-19,0.));
#21603=DIRECTION('ref_axis',(7.46735853138638E-19,1.,0.));
#21604=DIRECTION('',(-1.,0.,0.));
#21605=DIRECTION('center_axis',(1.,0.,0.));
#21606=DIRECTION('ref_axis',(0.,0.,1.));
#21607=DIRECTION('',(1.,0.,0.));
#21608=DIRECTION('center_axis',(1.,0.,0.));
#21609=DIRECTION('ref_axis',(0.,0.,-1.));
#21610=DIRECTION('',(-1.,0.,6.80579823082152E-36));
#21611=DIRECTION('',(-1.,0.,6.80579823082152E-36));
#21612=DIRECTION('center_axis',(1.,0.,0.));
#21613=DIRECTION('ref_axis',(0.,1.,0.));
#21614=DIRECTION('',(1.,0.,-6.80579823082152E-36));
#21615=DIRECTION('center_axis',(1.,-3.33478423293997E-20,0.));
#21616=DIRECTION('ref_axis',(-3.33478423293997E-20,-1.,0.));
#21617=DIRECTION('',(6.42769832910921E-36,1.92747052886312E-16,1.));
#21618=DIRECTION('',(-3.33478423293997E-20,-1.,2.04085114820801E-16));
#21619=DIRECTION('',(0.,0.,-1.));
#21620=DIRECTION('',(3.33478423293997E-20,1.,-2.31296463463574E-16));
#21621=DIRECTION('',(-8.08152366190323E-36,-2.43945488809238E-16,-1.));
#21622=DIRECTION('',(3.33478423293997E-20,1.,0.));
#21623=DIRECTION('center_axis',(7.71323799493105E-36,2.31296463463574E-16,
1.));
#21624=DIRECTION('ref_axis',(0.,-1.,2.31296463463574E-16));
#21625=DIRECTION('',(-1.,3.33478423293997E-20,0.));
#21626=DIRECTION('center_axis',(3.33478423293997E-20,1.,0.));
#21627=DIRECTION('ref_axis',(1.,-3.33478423293997E-20,0.));
#21628=DIRECTION('',(-1.,3.33478423293997E-20,0.));
#21629=DIRECTION('center_axis',(-6.80579823082151E-36,-2.04085114820801E-16,
-1.));
#21630=DIRECTION('ref_axis',(0.,-1.,2.04085114820801E-16));
#21631=DIRECTION('center_axis',(0.,-1.,0.));
#21632=DIRECTION('ref_axis',(0.,0.,-1.));
#21633=DIRECTION('',(-1.,0.,0.));
#21634=DIRECTION('',(-1.,0.,0.));
#21635=DIRECTION('center_axis',(-1.,0.,0.));
#21636=DIRECTION('ref_axis',(0.,0.,1.));
#21637=DIRECTION('',(0.,1.,0.));
#21638=DIRECTION('',(0.,1.,0.));
#21639=DIRECTION('center_axis',(0.,1.,0.));
#21640=DIRECTION('ref_axis',(1.,0.,0.));
#21641=DIRECTION('',(1.,0.,0.));
#21642=DIRECTION('',(1.,0.,0.));
#21643=DIRECTION('center_axis',(1.,0.,0.));
#21644=DIRECTION('ref_axis',(0.,1.,0.));
#21645=DIRECTION('',(0.,-1.,0.));
#21646=DIRECTION('',(0.,-1.,0.));
#21647=DIRECTION('center_axis',(0.,0.,-1.));
#21648=DIRECTION('ref_axis',(-1.,0.,0.));
#21649=DIRECTION('',(0.,0.,-1.));
#21650=DIRECTION('center_axis',(0.,0.,1.));
#21651=DIRECTION('ref_axis',(1.,0.,0.));
#21652=DIRECTION('center_axis',(0.,0.,-1.));
#21653=DIRECTION('ref_axis',(-1.,0.,0.));
#21654=DIRECTION('center_axis',(0.,0.,1.));
#21655=DIRECTION('ref_axis',(1.,0.,0.));
#21656=DIRECTION('',(0.,0.,-1.));
#21657=DIRECTION('center_axis',(0.,0.,1.));
#21658=DIRECTION('ref_axis',(1.,0.,0.));
#21659=DIRECTION('center_axis',(0.,0.,-1.));
#21660=DIRECTION('ref_axis',(-1.,0.,0.));
#21661=DIRECTION('',(0.,0.,-1.));
#21662=DIRECTION('center_axis',(0.,0.,1.));
#21663=DIRECTION('ref_axis',(1.,0.,0.));
#21664=DIRECTION('center_axis',(0.,0.,-1.));
#21665=DIRECTION('ref_axis',(-1.,0.,0.));
#21666=DIRECTION('',(0.,0.,-1.));
#21667=DIRECTION('center_axis',(0.,0.,1.));
#21668=DIRECTION('ref_axis',(1.,0.,0.));
#21669=DIRECTION('center_axis',(0.,0.,-1.));
#21670=DIRECTION('ref_axis',(-1.,0.,0.));
#21671=DIRECTION('',(0.,0.,-1.));
#21672=DIRECTION('center_axis',(0.,0.,1.));
#21673=DIRECTION('ref_axis',(1.,0.,0.));
#21674=DIRECTION('center_axis',(0.,0.,-1.));
#21675=DIRECTION('ref_axis',(-1.,0.,0.));
#21676=DIRECTION('center_axis',(0.,0.,1.));
#21677=DIRECTION('ref_axis',(1.,0.,0.));
#21678=DIRECTION('',(0.,0.,-1.));
#21679=DIRECTION('center_axis',(0.,0.,1.));
#21680=DIRECTION('ref_axis',(1.,0.,0.));
#21681=DIRECTION('center_axis',(0.,0.,-1.));
#21682=DIRECTION('ref_axis',(-1.,0.,0.));
#21683=DIRECTION('center_axis',(0.,0.,1.));
#21684=DIRECTION('ref_axis',(1.,0.,0.));
#21685=DIRECTION('',(0.,0.,-1.));
#21686=DIRECTION('center_axis',(0.,0.,1.));
#21687=DIRECTION('ref_axis',(1.,0.,0.));
#21688=DIRECTION('center_axis',(0.,0.,-1.));
#21689=DIRECTION('ref_axis',(-1.,0.,0.));
#21690=DIRECTION('',(0.,0.,-1.));
#21691=DIRECTION('center_axis',(0.,0.,1.));
#21692=DIRECTION('ref_axis',(1.,0.,0.));
#21693=DIRECTION('center_axis',(0.,0.,-1.));
#21694=DIRECTION('ref_axis',(-1.,0.,0.));
#21695=DIRECTION('',(0.,0.,-1.));
#21696=DIRECTION('center_axis',(0.,0.,1.));
#21697=DIRECTION('ref_axis',(1.,0.,0.));
#21698=DIRECTION('center_axis',(0.,0.,-1.));
#21699=DIRECTION('ref_axis',(-1.,0.,0.));
#21700=DIRECTION('',(0.,0.,-1.));
#21701=DIRECTION('center_axis',(0.,0.,1.));
#21702=DIRECTION('ref_axis',(1.,0.,0.));
#21703=DIRECTION('center_axis',(0.,0.,-1.));
#21704=DIRECTION('ref_axis',(-1.,0.,0.));
#21705=DIRECTION('',(0.,0.,-1.));
#21706=DIRECTION('center_axis',(0.,0.,1.));
#21707=DIRECTION('ref_axis',(1.,0.,0.));
#21708=DIRECTION('center_axis',(0.,0.,-1.));
#21709=DIRECTION('ref_axis',(-1.,0.,0.));
#21710=DIRECTION('',(0.,0.,-1.));
#21711=DIRECTION('center_axis',(0.,0.,1.));
#21712=DIRECTION('ref_axis',(1.,0.,0.));
#21713=DIRECTION('center_axis',(0.,0.,-1.));
#21714=DIRECTION('ref_axis',(-1.,0.,0.));
#21715=DIRECTION('',(0.,0.,-1.));
#21716=DIRECTION('center_axis',(0.,0.,1.));
#21717=DIRECTION('ref_axis',(1.,0.,0.));
#21718=DIRECTION('center_axis',(0.,0.,-1.));
#21719=DIRECTION('ref_axis',(-1.,0.,0.));
#21720=DIRECTION('',(0.,0.,-1.));
#21721=DIRECTION('center_axis',(0.,0.,1.));
#21722=DIRECTION('ref_axis',(1.,0.,0.));
#21723=DIRECTION('center_axis',(0.,0.,-1.));
#21724=DIRECTION('ref_axis',(-1.,0.,0.));
#21725=DIRECTION('',(0.,0.,-1.));
#21726=DIRECTION('center_axis',(0.,0.,1.));
#21727=DIRECTION('ref_axis',(1.,0.,0.));
#21728=DIRECTION('center_axis',(0.,0.,-1.));
#21729=DIRECTION('ref_axis',(-1.,0.,0.));
#21730=DIRECTION('',(0.,0.,-1.));
#21731=DIRECTION('center_axis',(0.,0.,1.));
#21732=DIRECTION('ref_axis',(1.,0.,0.));
#21733=DIRECTION('center_axis',(0.,-1.,0.));
#21734=DIRECTION('ref_axis',(0.,0.,-1.));
#21735=DIRECTION('',(-1.,0.,0.));
#21736=DIRECTION('',(0.,0.,-1.));
#21737=DIRECTION('',(-1.,0.,0.));
#21738=DIRECTION('',(0.,0.,-1.));
#21739=DIRECTION('center_axis',(-1.,0.,0.));
#21740=DIRECTION('ref_axis',(0.,0.,1.));
#21741=DIRECTION('',(0.,1.,0.));
#21742=DIRECTION('',(0.,1.,0.));
#21743=DIRECTION('',(0.,0.,-1.));
#21744=DIRECTION('center_axis',(1.57296039774614E-16,-1.,0.));
#21745=DIRECTION('ref_axis',(0.,0.,-1.));
#21746=DIRECTION('',(-1.,-1.57296039774614E-16,0.));
#21747=DIRECTION('',(-1.,-1.57296039774614E-16,0.));
#21748=DIRECTION('center_axis',(0.968859201920176,-0.247612291404526,0.));
#21749=DIRECTION('ref_axis',(0.,0.,-1.));
#21750=DIRECTION('',(-0.247612291404526,-0.968859201920176,0.));
#21751=DIRECTION('',(-0.247612291404526,-0.968859201920176,0.));
#21752=DIRECTION('',(0.,0.,-1.));
#21753=DIRECTION('center_axis',(0.,0.,-1.));
#21754=DIRECTION('ref_axis',(-1.,0.,0.));
#21755=DIRECTION('center_axis',(0.,0.,1.));
#21756=DIRECTION('ref_axis',(1.,0.,0.));
#21757=DIRECTION('center_axis',(0.,0.,1.));
#21758=DIRECTION('ref_axis',(1.,0.,0.));
#21759=DIRECTION('',(0.,0.,-1.));
#21760=DIRECTION('center_axis',(5.33319398640883E-16,-1.,0.));
#21761=DIRECTION('ref_axis',(0.,0.,-1.));
#21762=DIRECTION('',(-1.,-5.33319398640883E-16,0.));
#21763=DIRECTION('',(-1.,-5.33319398640883E-16,0.));
#21764=DIRECTION('center_axis',(0.662145231497846,-0.74937553496539,0.));
#21765=DIRECTION('ref_axis',(0.,0.,-1.));
#21766=DIRECTION('',(-0.74937553496539,-0.662145231497846,0.));
#21767=DIRECTION('',(-0.74937553496539,-0.662145231497846,0.));
#21768=DIRECTION('',(0.,0.,-1.));
#21769=DIRECTION('center_axis',(0.,0.,-1.));
#21770=DIRECTION('ref_axis',(-1.,0.,0.));
#21771=DIRECTION('center_axis',(0.,0.,1.));
#21772=DIRECTION('ref_axis',(1.,0.,0.));
#21773=DIRECTION('center_axis',(0.,0.,1.));
#21774=DIRECTION('ref_axis',(1.,0.,0.));
#21775=DIRECTION('',(0.,0.,-1.));
#21776=DIRECTION('center_axis',(0.,-1.,0.));
#21777=DIRECTION('ref_axis',(0.,0.,-1.));
#21778=DIRECTION('',(-1.,0.,0.));
#21779=DIRECTION('',(-1.,0.,0.));
#21780=DIRECTION('',(0.,0.,-1.));
#21781=DIRECTION('center_axis',(0.,0.,-1.));
#21782=DIRECTION('ref_axis',(-1.,0.,0.));
#21783=DIRECTION('center_axis',(0.,0.,1.));
#21784=DIRECTION('ref_axis',(1.,0.,0.));
#21785=DIRECTION('center_axis',(0.,0.,1.));
#21786=DIRECTION('ref_axis',(1.,0.,0.));
#21787=DIRECTION('',(0.,0.,-1.));
#21788=DIRECTION('center_axis',(-1.,-2.0289026509807E-16,0.));
#21789=DIRECTION('ref_axis',(-2.0289026509807E-16,1.,0.));
#21790=DIRECTION('',(-2.0289026509807E-16,1.,0.));
#21791=DIRECTION('',(-2.0289026509807E-16,1.,0.));
#21792=DIRECTION('',(0.,0.,-1.));
#21793=DIRECTION('center_axis',(0.,1.,0.));
#21794=DIRECTION('ref_axis',(1.,0.,0.));
#21795=DIRECTION('',(0.,0.,-1.));
#21796=DIRECTION('',(0.,0.,-1.));
#21797=DIRECTION('',(-1.,-1.98254111540206E-16,0.));
#21798=DIRECTION('',(1.,0.,0.));
#21799=DIRECTION('',(1.,0.,0.));
#21800=DIRECTION('',(0.,0.,-1.));
#21801=DIRECTION('center_axis',(1.,0.,0.));
#21802=DIRECTION('ref_axis',(0.,1.,0.));
#21803=DIRECTION('',(0.,0.,-1.));
#21804=DIRECTION('',(0.,-1.,0.));
#21805=DIRECTION('center_axis',(3.0952060520883E-16,-1.,0.));
#21806=DIRECTION('ref_axis',(0.,0.,-1.));
#21807=DIRECTION('',(0.,0.,-1.));
#21808=DIRECTION('',(-1.,-3.0952060520883E-16,0.));
#21809=DIRECTION('',(0.,0.,-1.));
#21810=DIRECTION('',(-1.,3.33478423293997E-20,0.));
#21811=DIRECTION('',(0.,0.,-1.));
#21812=DIRECTION('',(-1.,-1.0842021724855E-16,0.));
#21813=DIRECTION('center_axis',(1.,3.75567552354677E-14,0.));
#21814=DIRECTION('ref_axis',(-3.75567552354678E-14,1.,0.));
#21815=DIRECTION('',(3.75567552354677E-14,-1.,0.));
#21816=DIRECTION('',(3.75567552354677E-14,-1.,0.));
#21817=DIRECTION('',(0.,0.,-1.));
#21818=DIRECTION('center_axis',(0.,1.,0.));
#21819=DIRECTION('ref_axis',(1.,0.,0.));
#21820=DIRECTION('',(1.,0.,0.));
#21821=DIRECTION('',(1.,0.,0.));
#21822=DIRECTION('',(0.,0.,-1.));
#21823=DIRECTION('center_axis',(-1.,-1.25189184118226E-14,0.));
#21824=DIRECTION('ref_axis',(-1.25189184118226E-14,1.,0.));
#21825=DIRECTION('',(-1.25189184118226E-14,1.,0.));
#21826=DIRECTION('',(-1.25189184118226E-14,1.,0.));
#21827=DIRECTION('center_axis',(-1.,0.,0.));
#21828=DIRECTION('ref_axis',(0.,0.,1.));
#21829=DIRECTION('',(0.,1.,0.));
#21830=DIRECTION('center_axis',(1.,-7.46735853138638E-19,0.));
#21831=DIRECTION('ref_axis',(-7.46735853138638E-19,-1.,0.));
#21832=DIRECTION('',(-7.46735853138638E-19,-1.,0.));
#21833=DIRECTION('',(-7.46735853138638E-19,-1.,0.));
#21834=DIRECTION('center_axis',(0.,0.,1.));
#21835=DIRECTION('ref_axis',(1.,0.,0.));
#21836=DIRECTION('center_axis',(0.,0.,1.));
#21837=DIRECTION('ref_axis',(1.,0.,0.));
#21838=DIRECTION('center_axis',(7.71323799493105E-36,2.31296463463574E-16,
1.));
#21839=DIRECTION('ref_axis',(0.,-1.,2.31296463463574E-16));
#21840=DIRECTION('',(-1.,3.33478423293997E-20,0.));
#21841=DIRECTION('center_axis',(3.33478423293997E-20,1.,0.));
#21842=DIRECTION('ref_axis',(1.,-3.33478423293997E-20,0.));
#21843=DIRECTION('',(-1.,3.33478423293997E-20,0.));
#21844=DIRECTION('center_axis',(-6.80579823082151E-36,-2.04085114820801E-16,
-1.));
#21845=DIRECTION('ref_axis',(0.,-1.,2.04085114820801E-16));
#26841=CARTESIAN_POINT('',(0.,0.,0.));
#26842=CARTESIAN_POINT('Origin',(17.738300751771,49.437062129158,214.5));
#26843=CARTESIAN_POINT('',(13.738300751771,49.437062129158,214.5));
#26844=CARTESIAN_POINT('',(17.738300751771,53.437062129158,214.5));
#26845=CARTESIAN_POINT('Origin',(17.738300751771,49.437062129158,214.5));
#26846=CARTESIAN_POINT('',(13.738300751771,49.437062129158,212.5));
#26847=CARTESIAN_POINT('',(13.738300751771,49.437062129158,214.5));
#26848=CARTESIAN_POINT('',(17.738300751771,53.437062129158,212.5));
#26849=CARTESIAN_POINT('Origin',(17.738300751771,49.437062129158,212.5));
#26850=CARTESIAN_POINT('',(17.738300751771,53.437062129158,212.5));
#26851=CARTESIAN_POINT('Origin',(17.738300751771,35.437062129158,214.5));
#26852=CARTESIAN_POINT('',(17.738300751771,31.437062129158,214.5));
#26853=CARTESIAN_POINT('',(13.738300751771,35.437062129158,214.5));
#26854=CARTESIAN_POINT('Origin',(17.738300751771,35.437062129158,214.5));
#26855=CARTESIAN_POINT('',(17.738300751771,31.437062129158,212.5));
#26856=CARTESIAN_POINT('',(17.738300751771,31.437062129158,214.5));
#26857=CARTESIAN_POINT('',(13.738300751771,35.437062129158,212.5));
#26858=CARTESIAN_POINT('Origin',(17.738300751771,35.437062129158,212.5));
#26859=CARTESIAN_POINT('',(13.738300751771,35.437062129158,212.5));
#26860=CARTESIAN_POINT('Origin',(41.738300751771,35.437062129158,214.5));
#26861=CARTESIAN_POINT('',(45.738300751771,35.437062129158,214.5));
#26862=CARTESIAN_POINT('',(41.738300751771,31.437062129158,214.5));
#26863=CARTESIAN_POINT('Origin',(41.738300751771,35.437062129158,214.5));
#26864=CARTESIAN_POINT('',(45.738300751771,35.437062129158,212.5));
#26865=CARTESIAN_POINT('',(45.738300751771,35.437062129158,214.5));
#26866=CARTESIAN_POINT('',(41.738300751771,31.437062129158,212.5));
#26867=CARTESIAN_POINT('Origin',(41.738300751771,35.437062129158,212.5));
#26868=CARTESIAN_POINT('',(41.738300751771,31.437062129158,212.5));
#26869=CARTESIAN_POINT('Origin',(41.738300751771,49.437062129158,214.5));
#26870=CARTESIAN_POINT('',(41.738300751771,53.437062129158,214.5));
#26871=CARTESIAN_POINT('',(45.738300751771,49.437062129158,214.5));
#26872=CARTESIAN_POINT('Origin',(41.738300751771,49.437062129158,214.5));
#26873=CARTESIAN_POINT('',(41.738300751771,53.437062129158,212.5));
#26874=CARTESIAN_POINT('',(41.738300751771,53.437062129158,214.5));
#26875=CARTESIAN_POINT('',(45.738300751771,49.437062129158,212.5));
#26876=CARTESIAN_POINT('Origin',(41.738300751771,49.437062129158,212.5));
#26877=CARTESIAN_POINT('',(45.738300751771,49.437062129158,212.5));
#26878=CARTESIAN_POINT('Origin',(1.3592091877994,36.437062129158,214.5));
#26879=CARTESIAN_POINT('',(5.23464599548021,35.4466129635399,214.5));
#26880=CARTESIAN_POINT('',(1.3592091877994,32.437062129158,214.5));
#26881=CARTESIAN_POINT('Origin',(1.3592091877994,36.437062129158,214.5));
#26882=CARTESIAN_POINT('',(5.23464599548021,35.4466129635399,212.5));
#26883=CARTESIAN_POINT('',(5.23464599548021,35.4466129635399,214.5));
#26884=CARTESIAN_POINT('',(1.3592091877994,32.437062129158,212.5));
#26885=CARTESIAN_POINT('Origin',(1.3592091877994,36.437062129158,212.5));
#26886=CARTESIAN_POINT('',(1.3592091877994,32.437062129158,212.5));
#26887=CARTESIAN_POINT('Origin',(42.977211794544,76.437062129158,214.5));
#26888=CARTESIAN_POINT('',(45.625792720535,73.4395599892964,214.5));
#26889=CARTESIAN_POINT('',(42.977211794544,72.437062129158,214.5));
#26890=CARTESIAN_POINT('Origin',(42.977211794544,76.437062129158,214.5));
#26891=CARTESIAN_POINT('',(45.625792720535,73.4395599892964,212.5));
#26892=CARTESIAN_POINT('',(45.625792720535,73.4395599892964,214.5));
#26893=CARTESIAN_POINT('',(42.977211794544,72.437062129158,212.5));
#26894=CARTESIAN_POINT('Origin',(42.977211794544,76.437062129158,212.5));
#26895=CARTESIAN_POINT('',(42.977211794544,72.437062129158,212.5));
#26896=CARTESIAN_POINT('Origin',(-112.45844945829,-38.2430904326252,213.4));
#26897=CARTESIAN_POINT('',(-110.85844945829,-38.2430904326252,213.4));
#26898=CARTESIAN_POINT('',(-114.05844945829,-38.2430904326252,213.4));
#26899=CARTESIAN_POINT('Origin',(-112.45844945829,-38.2430904326252,213.4));
#26900=CARTESIAN_POINT('Origin',(-112.45844945829,-38.2430904326252,213.4));
#26901=CARTESIAN_POINT('',(-115.15844945829,-38.2430904326252,214.5));
#26902=CARTESIAN_POINT('',(-114.05844945829,-38.2430904326252,213.4));
#26903=CARTESIAN_POINT('Origin',(-112.45844945829,-38.2430904326252,214.5));
#26904=CARTESIAN_POINT('Origin',(-110.126903127,25.6553383360753,213.4));
#26905=CARTESIAN_POINT('',(-108.526903127,25.6553383360753,213.4));
#26906=CARTESIAN_POINT('',(-111.726903127,25.6553383360753,213.4));
#26907=CARTESIAN_POINT('Origin',(-110.126903127,25.6553383360753,213.4));
#26908=CARTESIAN_POINT('Origin',(-110.126903127,25.6553383360753,213.4));
#26909=CARTESIAN_POINT('',(-112.826903127,25.6553383360753,214.5));
#26910=CARTESIAN_POINT('',(-111.726903127,25.6553383360753,213.4));
#26911=CARTESIAN_POINT('Origin',(-110.126903127,25.6553383360753,214.5));
#26912=CARTESIAN_POINT('Origin',(-37.5407744425955,-7.8397685706167,213.4));
#26913=CARTESIAN_POINT('',(-35.9407744425954,-7.8397685706167,213.4));
#26914=CARTESIAN_POINT('',(-39.1407744425955,-7.8397685706167,213.4));
#26915=CARTESIAN_POINT('Origin',(-37.5407744425955,-7.8397685706167,213.4));
#26916=CARTESIAN_POINT('Origin',(-37.5407744425955,-7.8397685706167,213.4));
#26917=CARTESIAN_POINT('',(-40.2407744425955,-7.8397685706167,214.5));
#26918=CARTESIAN_POINT('',(-39.1407744425955,-7.8397685706167,213.4));
#26919=CARTESIAN_POINT('Origin',(-37.5407744425955,-7.8397685706167,214.5));
#26920=CARTESIAN_POINT('Origin',(40.4592255574045,-7.8397685706167,213.4));
#26921=CARTESIAN_POINT('',(42.0592255574045,-7.8397685706167,213.4));
#26922=CARTESIAN_POINT('',(38.8592255574045,-7.8397685706167,213.4));
#26923=CARTESIAN_POINT('Origin',(40.4592255574045,-7.8397685706167,213.4));
#26924=CARTESIAN_POINT('Origin',(40.4592255574045,-7.8397685706167,213.4));
#26925=CARTESIAN_POINT('',(37.7592255574045,-7.8397685706167,214.5));
#26926=CARTESIAN_POINT('',(38.8592255574045,-7.8397685706167,213.4));
#26927=CARTESIAN_POINT('Origin',(40.4592255574045,-7.8397685706167,214.5));
#26928=CARTESIAN_POINT('Origin',(73.324673000048,-35.1598100783688,213.4));
#26929=CARTESIAN_POINT('',(74.924673000048,-35.1598100783688,213.4));
#26930=CARTESIAN_POINT('',(71.724673000048,-35.1598100783688,213.4));
#26931=CARTESIAN_POINT('Origin',(73.324673000048,-35.1598100783688,213.4));
#26932=CARTESIAN_POINT('Origin',(73.324673000048,-35.1598100783688,213.4));
#26933=CARTESIAN_POINT('',(70.624673000048,-35.1598100783688,214.5));
#26934=CARTESIAN_POINT('',(71.724673000048,-35.1598100783688,213.4));
#26935=CARTESIAN_POINT('Origin',(73.324673000048,-35.1598100783688,214.5));
#26936=CARTESIAN_POINT('Origin',(54.6355073401705,34.895083038275,213.4));
#26937=CARTESIAN_POINT('',(56.2355073401705,34.895083038275,213.4));
#26938=CARTESIAN_POINT('',(53.0355073401705,34.895083038275,213.4));
#26939=CARTESIAN_POINT('Origin',(54.6355073401705,34.895083038275,213.4));
#26940=CARTESIAN_POINT('Origin',(54.6355073401705,34.895083038275,213.4));
#26941=CARTESIAN_POINT('',(51.9355073401705,34.895083038275,214.5));
#26942=CARTESIAN_POINT('',(53.0355073401705,34.895083038275,213.4));
#26943=CARTESIAN_POINT('Origin',(54.6355073401705,34.895083038275,214.5));
#26944=CARTESIAN_POINT('Origin',(5.7207051493956,10.2688129333875,213.4));
#26945=CARTESIAN_POINT('',(7.32070514939562,10.2688129333875,213.4));
#26946=CARTESIAN_POINT('',(4.1207051493956,10.2688129333875,213.4));
#26947=CARTESIAN_POINT('Origin',(5.7207051493956,10.2688129333875,213.4));
#26948=CARTESIAN_POINT('Origin',(5.7207051493956,10.2688129333875,213.4));
#26949=CARTESIAN_POINT('',(3.02070514939559,10.2688129333875,214.5));
#26950=CARTESIAN_POINT('',(4.1207051493956,10.2688129333875,213.4));
#26951=CARTESIAN_POINT('Origin',(5.7207051493956,10.2688129333875,214.5));
#26952=CARTESIAN_POINT('Origin',(77.738300751771,81.5680647192538,213.4));
#26953=CARTESIAN_POINT('',(79.338300751771,81.5680647192538,213.4));
#26954=CARTESIAN_POINT('',(76.138300751771,81.5680647192538,213.4));
#26955=CARTESIAN_POINT('Origin',(77.738300751771,81.5680647192538,213.4));
#26956=CARTESIAN_POINT('Origin',(77.738300751771,81.5680647192538,213.4));
#26957=CARTESIAN_POINT('',(75.038300751771,81.5680647192538,214.5));
#26958=CARTESIAN_POINT('',(76.138300751771,81.5680647192538,213.4));
#26959=CARTESIAN_POINT('Origin',(77.738300751771,81.5680647192538,214.5));
#26960=CARTESIAN_POINT('Origin',(39.747079812151,62.1619809501,213.4));
#26961=CARTESIAN_POINT('',(41.347079812151,62.1619809501,213.4));
#26962=CARTESIAN_POINT('',(38.147079812151,62.1619809501,213.4));
#26963=CARTESIAN_POINT('Origin',(39.747079812151,62.1619809501,213.4));
#26964=CARTESIAN_POINT('Origin',(39.747079812151,62.1619809501,213.4));
#26965=CARTESIAN_POINT('',(37.047079812151,62.1619809501,214.5));
#26966=CARTESIAN_POINT('',(38.147079812151,62.1619809501,213.4));
#26967=CARTESIAN_POINT('Origin',(39.747079812151,62.1619809501,214.5));
#26968=CARTESIAN_POINT('Origin',(25.1879034811638,63.7619809501,213.4));
#26969=CARTESIAN_POINT('',(27.287903481164,63.7619809501,213.4));
#26970=CARTESIAN_POINT('',(23.0879034811638,63.7619809501,213.4));
#26971=CARTESIAN_POINT('Origin',(25.1879034811638,63.7619809501,213.4));
#26972=CARTESIAN_POINT('Origin',(25.1879034811638,63.7619809501,213.4));
#26973=CARTESIAN_POINT('',(21.9879034811638,63.7619809501,214.5));
#26974=CARTESIAN_POINT('',(23.0879034811638,63.7619809501,213.4));
#26975=CARTESIAN_POINT('Origin',(25.1879034811638,63.7619809501,214.5));
#26976=CARTESIAN_POINT('Origin',(-55.2792948506043,10.2688129333875,213.4));
#26977=CARTESIAN_POINT('',(-53.6792948506043,10.2688129333875,213.4));
#26978=CARTESIAN_POINT('',(-56.8792948506043,10.2688129333875,213.4));
#26979=CARTESIAN_POINT('Origin',(-55.2792948506043,10.2688129333875,213.4));
#26980=CARTESIAN_POINT('Origin',(-55.2792948506043,10.2688129333875,213.4));
#26981=CARTESIAN_POINT('',(-57.9792948506043,10.2688129333875,214.5));
#26982=CARTESIAN_POINT('',(-56.8792948506043,10.2688129333875,213.4));
#26983=CARTESIAN_POINT('Origin',(-55.2792948506043,10.2688129333875,214.5));
#26984=CARTESIAN_POINT('Origin',(-11.261699248229,29.437062129158,213.4));
#26985=CARTESIAN_POINT('',(-9.66169924822899,29.437062129158,213.4));
#26986=CARTESIAN_POINT('',(-12.861699248229,29.437062129158,213.4));
#26987=CARTESIAN_POINT('Origin',(-11.261699248229,29.437062129158,213.4));
#26988=CARTESIAN_POINT('Origin',(-11.261699248229,29.437062129158,213.4));
#26989=CARTESIAN_POINT('',(-13.961699248229,29.437062129158,214.5));
#26990=CARTESIAN_POINT('',(-12.861699248229,29.437062129158,213.4));
#26991=CARTESIAN_POINT('Origin',(-11.261699248229,29.437062129158,214.5));
#26992=CARTESIAN_POINT('Origin',(-65.261699248229,29.437062129158,213.4));
#26993=CARTESIAN_POINT('',(-63.661699248229,29.437062129158,213.4));
#26994=CARTESIAN_POINT('',(-66.861699248229,29.437062129158,213.4));
#26995=CARTESIAN_POINT('Origin',(-65.261699248229,29.437062129158,213.4));
#26996=CARTESIAN_POINT('Origin',(-65.261699248229,29.437062129158,213.4));
#26997=CARTESIAN_POINT('',(-67.961699248229,29.437062129158,214.5));
#26998=CARTESIAN_POINT('',(-66.861699248229,29.437062129158,213.4));
#26999=CARTESIAN_POINT('Origin',(-65.261699248229,29.437062129158,214.5));
#27000=CARTESIAN_POINT('Origin',(-123.261699248229,-48.562937870842,210.5));
#27001=CARTESIAN_POINT('',(57.335333187315,-46.562937870842,210.5));
#27002=CARTESIAN_POINT('',(57.335333187315,-48.562937870842,210.5));
#27003=CARTESIAN_POINT('',(57.335333187315,-48.562937870842,210.5));
#27004=CARTESIAN_POINT('',(67.799693512506,-48.562937870842,210.5));
#27005=CARTESIAN_POINT('',(57.335333187315,-48.562937870842,210.5));
#27006=CARTESIAN_POINT('',(67.799693512506,-46.562937870842,210.5));
#27007=CARTESIAN_POINT('',(67.799693512506,-48.562937870842,210.5));
#27008=CARTESIAN_POINT('',(57.335333187315,-46.562937870842,210.5));
#27009=CARTESIAN_POINT('Origin',(-88.261699248229,-31.562937870842,251.410152916687));
#27010=CARTESIAN_POINT('',(-88.261699248229,-47.762937870842,194.5));
#27011=CARTESIAN_POINT('',(-88.261699248229,-48.562937870842,195.3));
#27012=CARTESIAN_POINT('Origin',(-88.261699248229,-47.762937870842,195.3));
#27013=CARTESIAN_POINT('',(-88.261699248229,-48.562937870842,212.5));
#27014=CARTESIAN_POINT('',(-88.261699248229,-48.562937870842,251.410152916687));
#27015=CARTESIAN_POINT('',(-88.261699248229,-45.7629378708421,212.5));
#27016=CARTESIAN_POINT('',(-88.261699248229,-31.562937870842,212.5));
#27017=CARTESIAN_POINT('',(-88.261699248229,-46.5629378708421,211.7));
#27018=CARTESIAN_POINT('Origin',(-88.261699248229,-45.7629378708421,211.7));
#27019=CARTESIAN_POINT('',(-88.261699248229,-46.562937870842,197.3));
#27020=CARTESIAN_POINT('',(-88.261699248229,-46.562937870842,214.5));
#27021=CARTESIAN_POINT('',(-88.261699248229,-45.762937870842,196.5));
#27022=CARTESIAN_POINT('Origin',(-88.261699248229,-45.762937870842,197.3));
#27023=CARTESIAN_POINT('',(-88.261699248229,-31.562937870842,196.5));
#27024=CARTESIAN_POINT('',(-88.261699248229,-46.5629378708419,196.5));
#27025=CARTESIAN_POINT('',(-88.261699248229,-31.562937870842,194.5));
#27026=CARTESIAN_POINT('',(-88.261699248229,-31.562937870842,251.410152916687));
#27027=CARTESIAN_POINT('',(-88.261699248229,-31.562937870842,194.5));
#27028=CARTESIAN_POINT('Origin',(-123.261699248229,-48.562937870842,196.5));
#27029=CARTESIAN_POINT('',(-33.261699248229,-45.762937870842,196.5));
#27030=CARTESIAN_POINT('',(-23.261699248229,-45.762937870842,196.5));
#27031=CARTESIAN_POINT('',(76.738300751771,-45.762937870842,196.5));
#27032=CARTESIAN_POINT('',(-23.261699248229,-47.762937870842,196.5));
#27033=CARTESIAN_POINT('',(-23.261699248229,-47.762937870842,196.5));
#27034=CARTESIAN_POINT('',(-33.261699248229,-47.762937870842,196.5));
#27035=CARTESIAN_POINT('',(-33.261699248229,-47.762937870842,196.5));
#27036=CARTESIAN_POINT('',(-33.261699248229,-31.562937870842,196.5));
#27037=CARTESIAN_POINT('Origin',(-23.261699248229,-47.762937870842,196.5));
#27038=CARTESIAN_POINT('',(-23.261699248229,-31.562937870842,194.5));
#27039=CARTESIAN_POINT('',(-23.261699248229,-47.762937870842,194.5));
#27040=CARTESIAN_POINT('',(-23.261699248229,-47.762937870842,194.5));
#27041=CARTESIAN_POINT('',(-23.261699248229,-47.762937870842,196.5));
#27042=CARTESIAN_POINT('',(-23.261699248229,-31.562937870842,196.5));
#27043=CARTESIAN_POINT('',(-23.261699248229,-47.762937870842,196.5));
#27044=CARTESIAN_POINT('',(-23.261699248229,-31.562937870842,196.5));
#27045=CARTESIAN_POINT('Origin',(-33.261699248229,-47.762937870842,196.5));
#27046=CARTESIAN_POINT('',(-33.261699248229,-47.762937870842,194.5));
#27047=CARTESIAN_POINT('',(-33.261699248229,-47.762937870842,194.5));
#27048=CARTESIAN_POINT('',(-33.261699248229,-47.762937870842,196.5));
#27049=CARTESIAN_POINT('Origin',(-33.261699248229,-31.562937870842,196.5));
#27050=CARTESIAN_POINT('',(-33.261699248229,-31.562937870842,194.5));
#27051=CARTESIAN_POINT('',(-33.261699248229,-31.562937870842,194.5));
#27052=CARTESIAN_POINT('',(-33.261699248229,-31.562937870842,196.5));
#27053=CARTESIAN_POINT('',(-33.261699248229,-31.562937870842,196.5));
#27054=CARTESIAN_POINT('',(-33.261699248229,-31.562937870842,196.5));
#27055=CARTESIAN_POINT('Origin',(82.241473619047,-45.762937870842,211.7));
#27056=CARTESIAN_POINT('',(53.335333187315,-46.562937870842,211.7));
#27057=CARTESIAN_POINT('',(53.335333187315,-46.562937870842,211.7));
#27058=CARTESIAN_POINT('',(53.335333187315,-45.762937870842,212.5));
#27059=CARTESIAN_POINT('',(-123.261699248229,-45.7629378708421,212.5));
#27060=CARTESIAN_POINT('Origin',(53.335333187315,-45.762937870842,211.7));
#27061=CARTESIAN_POINT('Origin',(70.6019681378195,-45.762937870842,197.3));
#27062=CARTESIAN_POINT('',(76.738300751771,-45.762937870842,196.5));
#27063=CARTESIAN_POINT('',(76.738300751771,-46.562937870842,197.3));
#27064=CARTESIAN_POINT('',(70.6019681378195,-46.562937870842,197.3));
#27065=CARTESIAN_POINT('',(76.738300751771,-45.762937870842,196.5));
#27066=CARTESIAN_POINT('Origin',(76.738300751771,-45.762937870842,197.3));
#27067=CARTESIAN_POINT('',(76.738300751771,-45.762937870842,196.5));
#27068=CARTESIAN_POINT('Origin',(82.241473619047,-47.762937870842,213.7));
#27069=CARTESIAN_POINT('',(-123.261699248229,-48.562937870842,213.7));
#27070=CARTESIAN_POINT('',(-123.261699248229,-47.762937870842,214.5));
#27071=CARTESIAN_POINT('Origin',(-123.261699248229,-47.762937870842,213.7));
#27072=CARTESIAN_POINT('',(57.335333187315,-48.562937870842,213.7));
#27073=CARTESIAN_POINT('',(-123.261699248229,-48.562937870842,213.7));
#27074=CARTESIAN_POINT('',(57.335333187315,-47.762937870842,214.5));
#27075=CARTESIAN_POINT('Origin',(57.335333187315,-47.762937870842,213.7));
#27076=CARTESIAN_POINT('',(57.335333187315,-47.762937870842,214.5));
#27077=CARTESIAN_POINT('Origin',(76.738300751771,-47.762937870842,195.3));
#27078=CARTESIAN_POINT('',(-123.261699248229,-47.762937870842,194.5));
#27079=CARTESIAN_POINT('',(76.738300751771,-47.762937870842,194.5));
#27080=CARTESIAN_POINT('',(-123.261699248229,-47.762937870842,194.5));
#27081=CARTESIAN_POINT('',(76.738300751771,-48.562937870842,195.3));
#27082=CARTESIAN_POINT('Origin',(76.738300751771,-47.762937870842,195.3));
#27083=CARTESIAN_POINT('',(76.738300751771,-48.562937870842,195.3));
#27084=CARTESIAN_POINT('Origin',(76.738300751771,-48.562937870842,212.5));
#27085=CARTESIAN_POINT('',(76.738300751771,-48.562937870842,212.5));
#27086=CARTESIAN_POINT('',(76.738300751771,-48.562937870842,212.5));
#27087=CARTESIAN_POINT('',(76.738300751771,-31.562937870842,194.5));
#27088=CARTESIAN_POINT('',(76.738300751771,-31.562937870842,194.5));
#27089=CARTESIAN_POINT('',(76.738300751771,-31.562937870842,196.5));
#27090=CARTESIAN_POINT('',(76.738300751771,-31.562937870842,196.5));
#27091=CARTESIAN_POINT('',(76.738300751771,-46.562937870842,196.5));
#27092=CARTESIAN_POINT('',(76.738300751771,-46.562937870842,212.5));
#27093=CARTESIAN_POINT('',(76.738300751771,-46.562937870842,212.5));
#27094=CARTESIAN_POINT('',(76.738300751771,-46.562937870842,212.5));
#27095=CARTESIAN_POINT('Origin',(76.738300751771,-46.562937870842,196.5));
#27096=CARTESIAN_POINT('',(76.738300751771,-31.562937870842,196.5));
#27097=CARTESIAN_POINT('Origin',(76.738300751771,-31.562937870842,196.5));
#27098=CARTESIAN_POINT('',(76.738300751771,-31.562937870842,194.5));
#27099=CARTESIAN_POINT('Origin',(76.738300751771,-31.562937870842,194.5));
#27100=CARTESIAN_POINT('Origin',(13.738300751771,53.437062129158,214.5));
#27101=CARTESIAN_POINT('',(13.738300751771,53.437062129158,212.5));
#27102=CARTESIAN_POINT('',(13.738300751771,53.437062129158,214.5));
#27103=CARTESIAN_POINT('Origin',(45.738300751771,53.437062129158,214.5));
#27104=CARTESIAN_POINT('',(45.738300751771,53.437062129158,214.5));
#27105=CARTESIAN_POINT('',(45.738300751771,53.437062129158,212.5));
#27106=CARTESIAN_POINT('Origin',(13.738300751771,31.437062129158,214.5));
#27107=CARTESIAN_POINT('',(13.738300751771,31.437062129158,214.5));
#27108=CARTESIAN_POINT('',(13.738300751771,31.437062129158,212.5));
#27109=CARTESIAN_POINT('Origin',(13.738300751771,53.437062129158,214.5));
#27110=CARTESIAN_POINT('',(13.738300751771,53.437062129158,214.5));
#27111=CARTESIAN_POINT('',(13.738300751771,53.437062129158,212.5));
#27112=CARTESIAN_POINT('Origin',(-65.261699248229,29.437062129158,214.5));
#27113=CARTESIAN_POINT('',(-63.661699248229,29.437062129158,212.5));
#27114=CARTESIAN_POINT('',(-63.661699248229,29.437062129158,214.5));
#27115=CARTESIAN_POINT('Origin',(-65.261699248229,29.437062129158,212.5));
#27116=CARTESIAN_POINT('Origin',(65.445980708565,16.608649616242,214.5));
#27117=CARTESIAN_POINT('',(66.6006799111879,16.608649616242,214.5));
#27118=CARTESIAN_POINT('Origin',(65.445980708565,16.608649616242,214.5));
#27119=CARTESIAN_POINT('',(66.6006799111879,16.608649616242,212.5));
#27120=CARTESIAN_POINT('',(66.6006799111879,16.608649616242,214.5));
#27121=CARTESIAN_POINT('Origin',(65.445980708565,16.608649616242,212.5));
#27122=CARTESIAN_POINT('Origin',(-55.2792948506043,10.2688129333875,214.5));
#27123=CARTESIAN_POINT('',(-53.6792948506043,10.2688129333875,212.5));
#27124=CARTESIAN_POINT('',(-53.6792948506043,10.2688129333875,214.5));
#27125=CARTESIAN_POINT('Origin',(-55.2792948506043,10.2688129333875,212.5));
#27126=CARTESIAN_POINT('Origin',(5.7207051493956,10.2688129333875,214.5));
#27127=CARTESIAN_POINT('',(7.3207051493956,10.2688129333875,212.5));
#27128=CARTESIAN_POINT('',(7.3207051493956,10.2688129333875,214.5));
#27129=CARTESIAN_POINT('Origin',(5.7207051493956,10.2688129333875,212.5));
#27130=CARTESIAN_POINT('Origin',(-11.261699248229,29.437062129158,214.5));
#27131=CARTESIAN_POINT('',(-9.66169924822899,29.437062129158,212.5));
#27132=CARTESIAN_POINT('',(-9.66169924822899,29.437062129158,214.5));
#27133=CARTESIAN_POINT('Origin',(-11.261699248229,29.437062129158,212.5));
#27134=CARTESIAN_POINT('Origin',(-5.54425899443339,28.0125156091345,214.5));
#27135=CARTESIAN_POINT('',(-4.21104341383355,28.0125156091345,214.5));
#27136=CARTESIAN_POINT('Origin',(-5.54425899443339,28.0125156091345,214.5));
#27137=CARTESIAN_POINT('',(-4.21104341383355,28.0125156091345,212.5));
#27138=CARTESIAN_POINT('',(-4.21104341383355,28.0125156091345,214.5));
#27139=CARTESIAN_POINT('Origin',(-5.54425899443339,28.0125156091345,212.5));
#27140=CARTESIAN_POINT('Origin',(-1.6080987088528,28.0125156091345,214.5));
#27141=CARTESIAN_POINT('',(-0.287031131713716,28.0125156091345,214.5));
#27142=CARTESIAN_POINT('Origin',(-1.6080987088528,28.0125156091345,214.5));
#27143=CARTESIAN_POINT('',(-0.287031131713716,28.0125156091345,212.5));
#27144=CARTESIAN_POINT('',(-0.287031131713716,28.0125156091345,214.5));
#27145=CARTESIAN_POINT('Origin',(-1.6080987088528,28.0125156091345,212.5));
#27146=CARTESIAN_POINT('Origin',(25.1879034811638,63.7619809501,214.5));
#27147=CARTESIAN_POINT('',(27.2879034811638,63.7619809501,212.5));
#27148=CARTESIAN_POINT('',(27.2879034811638,63.7619809501,214.5));
#27149=CARTESIAN_POINT('Origin',(25.1879034811638,63.7619809501,212.5));
#27150=CARTESIAN_POINT('Origin',(54.6355073401705,34.895083038275,214.5));
#27151=CARTESIAN_POINT('',(56.2355073401705,34.895083038275,212.5));
#27152=CARTESIAN_POINT('',(56.2355073401705,34.895083038275,214.5));
#27153=CARTESIAN_POINT('Origin',(54.6355073401705,34.895083038275,212.5));
#27154=CARTESIAN_POINT('Origin',(39.747079812151,62.1619809501,214.5));
#27155=CARTESIAN_POINT('',(41.347079812151,62.1619809501,212.5));
#27156=CARTESIAN_POINT('',(41.347079812151,62.1619809501,214.5));
#27157=CARTESIAN_POINT('Origin',(39.747079812151,62.1619809501,212.5));
#27158=CARTESIAN_POINT('Origin',(77.738300751771,81.5680647192538,214.5));
#27159=CARTESIAN_POINT('',(79.338300751771,81.5680647192538,212.5));
#27160=CARTESIAN_POINT('',(79.338300751771,81.5680647192538,214.5));
#27161=CARTESIAN_POINT('Origin',(77.738300751771,81.5680647192538,212.5));
#27162=CARTESIAN_POINT('Origin',(73.324673000048,-35.1598100783688,214.5));
#27163=CARTESIAN_POINT('',(74.924673000048,-35.1598100783688,212.5));
#27164=CARTESIAN_POINT('',(74.924673000048,-35.1598100783688,214.5));
#27165=CARTESIAN_POINT('Origin',(73.324673000048,-35.1598100783688,212.5));
#27166=CARTESIAN_POINT('Origin',(40.4592255574045,-7.8397685706167,214.5));
#27167=CARTESIAN_POINT('',(42.0592255574045,-7.8397685706167,212.5));
#27168=CARTESIAN_POINT('',(42.0592255574045,-7.8397685706167,214.5));
#27169=CARTESIAN_POINT('Origin',(40.4592255574045,-7.8397685706167,212.5));
#27170=CARTESIAN_POINT('Origin',(-37.5407744425955,-7.8397685706167,214.5));
#27171=CARTESIAN_POINT('',(-35.9407744425955,-7.8397685706167,212.5));
#27172=CARTESIAN_POINT('',(-35.9407744425955,-7.8397685706167,214.5));
#27173=CARTESIAN_POINT('Origin',(-37.5407744425955,-7.8397685706167,212.5));
#27174=CARTESIAN_POINT('Origin',(-112.45844945829,-38.2430904326252,214.5));
#27175=CARTESIAN_POINT('',(-110.85844945829,-38.2430904326252,212.5));
#27176=CARTESIAN_POINT('',(-110.85844945829,-38.2430904326252,214.5));
#27177=CARTESIAN_POINT('Origin',(-112.45844945829,-38.2430904326252,212.5));
#27178=CARTESIAN_POINT('Origin',(-110.126903127,25.6553383360753,214.5));
#27179=CARTESIAN_POINT('',(-108.526903127,25.6553383360753,212.5));
#27180=CARTESIAN_POINT('',(-108.526903127,25.6553383360753,214.5));
#27181=CARTESIAN_POINT('Origin',(-110.126903127,25.6553383360753,212.5));
#27182=CARTESIAN_POINT('Origin',(-83.761699248229,33.437062129158,214.5));
#27183=CARTESIAN_POINT('',(-83.761699248229,33.437062129158,212.5));
#27184=CARTESIAN_POINT('',(-123.261699248229,33.437062129158,212.5));
#27185=CARTESIAN_POINT('',(-83.761699248229,33.437062129158,212.5));
#27186=CARTESIAN_POINT('',(-123.261699248229,33.437062129158,214.5));
#27187=CARTESIAN_POINT('',(-123.261699248229,33.437062129158,214.5));
#27188=CARTESIAN_POINT('',(-83.761699248229,33.437062129158,214.5));
#27189=CARTESIAN_POINT('',(-83.761699248229,33.437062129158,214.5));
#27190=CARTESIAN_POINT('',(-83.761699248229,33.437062129158,214.5));
#27191=CARTESIAN_POINT('Origin',(-83.761699248229,32.437062129158,214.5));
#27192=CARTESIAN_POINT('',(-83.761699248229,32.437062129158,212.5));
#27193=CARTESIAN_POINT('',(-83.761699248229,32.437062129158,212.5));
#27194=CARTESIAN_POINT('',(-83.761699248229,32.437062129158,214.5));
#27195=CARTESIAN_POINT('',(-83.761699248229,32.437062129158,214.5));
#27196=CARTESIAN_POINT('',(-83.761699248229,32.437062129158,214.5));
#27197=CARTESIAN_POINT('Origin',(4.46549215277239,32.437062129158,214.5));
#27198=CARTESIAN_POINT('',(4.46549215277239,32.437062129158,214.5));
#27199=CARTESIAN_POINT('',(4.46549215277239,32.437062129158,212.5));
#27200=CARTESIAN_POINT('Origin',(13.5853385358292,68.121264388277,214.5));
#27201=CARTESIAN_POINT('',(13.5853385358292,68.121264388277,212.5));
#27202=CARTESIAN_POINT('',(13.5853385358292,68.121264388277,212.5));
#27203=CARTESIAN_POINT('',(13.5853385358292,68.121264388277,214.5));
#27204=CARTESIAN_POINT('',(13.5853385358292,68.121264388277,214.5));
#27205=CARTESIAN_POINT('',(13.5853385358292,68.121264388277,214.5));
#27206=CARTESIAN_POINT('Origin',(20.3202472047774,65.4209130265812,214.5));
#27207=CARTESIAN_POINT('',(18.4696948477504,72.437062129158,212.5));
#27208=CARTESIAN_POINT('Origin',(20.3202472047774,65.4209130265812,212.5));
#27209=CARTESIAN_POINT('',(18.4696948477504,72.437062129158,214.5));
#27210=CARTESIAN_POINT('Origin',(20.3202472047774,65.4209130265812,214.5));
#27211=CARTESIAN_POINT('',(18.4696948477504,72.437062129158,214.5));
#27212=CARTESIAN_POINT('Origin',(44.4912268662385,72.437062129158,214.5));
#27213=CARTESIAN_POINT('',(44.4912268662385,72.437062129158,214.5));
#27214=CARTESIAN_POINT('',(44.4912268662385,72.437062129158,212.5));
#27215=CARTESIAN_POINT('Origin',(66.7028317907535,92.0631475809084,214.5));
#27216=CARTESIAN_POINT('',(66.7028317907535,92.0631475809084,212.5));
#27217=CARTESIAN_POINT('',(66.7028317907535,92.0631475809084,212.5));
#27218=CARTESIAN_POINT('',(66.7028317907535,92.0631475809084,214.5));
#27219=CARTESIAN_POINT('',(66.7028317907535,92.0631475809084,214.5));
#27220=CARTESIAN_POINT('',(66.7028317907535,92.0631475809084,214.5));
#27221=CARTESIAN_POINT('Origin',(72.526950809562,86.133283776482,214.5));
#27222=CARTESIAN_POINT('',(72.1651329632355,94.437062129158,212.5));
#27223=CARTESIAN_POINT('Origin',(72.526950809562,86.133283776482,212.5));
#27224=CARTESIAN_POINT('',(72.1651329632355,94.437062129158,214.5));
#27225=CARTESIAN_POINT('Origin',(72.526950809562,86.133283776482,214.5));
#27226=CARTESIAN_POINT('',(72.1651329632355,94.437062129158,214.5));
#27227=CARTESIAN_POINT('Origin',(82.712821075816,94.437062129158,214.5));
#27228=CARTESIAN_POINT('',(82.712821075816,94.437062129158,212.5));
#27229=CARTESIAN_POINT('',(82.712821075816,94.437062129158,212.5));
#27230=CARTESIAN_POINT('',(82.712821075816,94.437062129158,214.5));
#27231=CARTESIAN_POINT('',(82.712821075816,94.437062129158,214.5));
#27232=CARTESIAN_POINT('',(82.712821075816,94.437062129158,214.5));
#27233=CARTESIAN_POINT('Origin',(82.241473619047,86.8223151727852,214.5));
#27234=CARTESIAN_POINT('',(89.738300751771,88.2379855357732,212.5));
#27235=CARTESIAN_POINT('Origin',(82.241473619047,86.8223151727852,212.5));
#27236=CARTESIAN_POINT('',(89.738300751771,88.2379855357732,214.5));
#27237=CARTESIAN_POINT('Origin',(82.241473619047,86.8223151727852,214.5));
#27238=CARTESIAN_POINT('',(89.738300751771,88.2379855357732,214.5));
#27239=CARTESIAN_POINT('Origin',(89.738300751771,-48.562937870842,214.5));
#27240=CARTESIAN_POINT('',(89.738300751771,-48.562937870842,212.5));
#27241=CARTESIAN_POINT('',(89.738300751771,-48.562937870842,212.5));
#27242=CARTESIAN_POINT('',(89.738300751771,-48.562937870842,214.5));
#27243=CARTESIAN_POINT('',(89.738300751771,-48.562937870842,214.5));
#27244=CARTESIAN_POINT('',(89.738300751771,-48.562937870842,214.5));
#27245=CARTESIAN_POINT('Origin',(67.799693512506,-48.562937870842,214.5));
#27246=CARTESIAN_POINT('',(57.335333187315,-48.562937870842,214.5));
#27247=CARTESIAN_POINT('',(-123.261699248229,-48.562937870842,212.5));
#27248=CARTESIAN_POINT('',(-123.261699248229,-48.562937870842,214.5));
#27249=CARTESIAN_POINT('',(-123.261699248229,-48.562937870842,212.5));
#27250=CARTESIAN_POINT('',(67.799693512506,-48.562937870842,212.5));
#27251=CARTESIAN_POINT('',(67.799693512506,-48.562937870842,214.5));
#27252=CARTESIAN_POINT('',(67.799693512506,-48.562937870842,214.5));
#27253=CARTESIAN_POINT('',(67.799693512506,-48.562937870842,214.5));
#27254=CARTESIAN_POINT('Origin',(67.799693512506,-46.562937870842,214.5));
#27255=CARTESIAN_POINT('',(67.799693512506,-46.562937870842,214.5));
#27256=CARTESIAN_POINT('',(67.799693512506,-46.562937870842,214.5));
#27257=CARTESIAN_POINT('',(67.799693512506,-46.562937870842,214.5));
#27258=CARTESIAN_POINT('Origin',(70.6019681378195,-46.562937870842,214.5));
#27259=CARTESIAN_POINT('',(57.335333187315,-46.562937870842,214.5));
#27260=CARTESIAN_POINT('',(57.335333187315,-46.562937870842,214.5));
#27261=CARTESIAN_POINT('',(70.6019681378195,-46.562937870842,214.5));
#27262=CARTESIAN_POINT('',(70.6019681378195,-46.562937870842,214.5));
#27263=CARTESIAN_POINT('',(70.6019681378195,-46.562937870842,212.5));
#27264=CARTESIAN_POINT('',(70.6019681378195,-46.562937870842,214.5));
#27265=CARTESIAN_POINT('',(76.738300751771,-46.562937870842,212.5));
#27266=CARTESIAN_POINT('',(53.335333187315,-46.562937870842,214.5));
#27267=CARTESIAN_POINT('',(53.335333187315,-46.562937870842,214.5));
#27268=CARTESIAN_POINT('',(57.335333187315,-46.562937870842,214.5));
#27269=CARTESIAN_POINT('Origin',(70.6019681378195,-44.3458473281465,214.5));
#27270=CARTESIAN_POINT('',(70.6019681378195,-44.3458473281465,212.5));
#27271=CARTESIAN_POINT('',(70.6019681378195,-44.3458473281465,212.5));
#27272=CARTESIAN_POINT('',(70.6019681378195,-44.3458473281465,214.5));
#27273=CARTESIAN_POINT('',(70.6019681378195,-44.3458473281465,214.5));
#27274=CARTESIAN_POINT('',(70.6019681378195,-44.3458473281465,214.5));
#27275=CARTESIAN_POINT('Origin',(53.335333187315,-44.3458473281465,214.5));
#27276=CARTESIAN_POINT('',(53.335333187315,-44.3458473281465,212.5));
#27277=CARTESIAN_POINT('',(53.335333187315,-44.3458473281465,212.5));
#27278=CARTESIAN_POINT('',(53.335333187315,-44.3458473281465,214.5));
#27279=CARTESIAN_POINT('',(53.335333187315,-44.3458473281465,214.5));
#27280=CARTESIAN_POINT('',(53.335333187315,-44.3458473281465,214.5));
#27281=CARTESIAN_POINT('Origin',(53.335333187315,-46.562937870842,214.5));
#27282=CARTESIAN_POINT('',(53.335333187315,-46.562937870842,212.5));
#27283=CARTESIAN_POINT('',(53.335333187315,-46.562937870842,214.5));
#27284=CARTESIAN_POINT('Origin',(57.335333187315,-48.562937870842,214.5));
#27285=CARTESIAN_POINT('',(57.335333187315,-48.562937870842,214.5));
#27286=CARTESIAN_POINT('Origin',(-123.261699248229,33.437062129158,214.5));
#27287=CARTESIAN_POINT('',(-123.261699248229,33.437062129158,212.5));
#27288=CARTESIAN_POINT('',(-123.261699248229,33.437062129158,214.5));
#27289=CARTESIAN_POINT('Origin',(82.241473619047,86.8223151727852,212.5));
#27290=CARTESIAN_POINT('Origin',(82.241473619047,86.8223151727852,214.5));
#27291=CARTESIAN_POINT('Origin',(76.738300751771,-46.562937870842,196.5));
#27292=CARTESIAN_POINT('',(76.738300751771,-31.562937870842,196.5));
#27293=CARTESIAN_POINT('Origin',(76.738300751771,-31.562937870842,196.5));
#27294=CARTESIAN_POINT('',(76.738300751771,-31.562937870842,194.5));
#27295=CARTESIAN_POINT('Origin',(76.738300751771,-31.562937870842,194.5));
#36649=UNCERTAINTY_MEASURE_WITH_UNIT(LENGTH_MEASURE(0.01),#36669,
'DISTANCE_ACCURACY_VALUE',
'Maximum model space distance between geometric entities at asserted c
onnectivities');
#36656=UNCERTAINTY_MEASURE_WITH_UNIT(LENGTH_MEASURE(0.01),#36669,
'DISTANCE_ACCURACY_VALUE',
'Maximum model space distance between geometric entities at asserted c
onnectivities');
#36661=(
GEOMETRIC_REPRESENTATION_CONTEXT(3)
GLOBAL_UNCERTAINTY_ASSIGNED_CONTEXT((#36649))
GLOBAL_UNIT_ASSIGNED_CONTEXT((#36669,#36671,#36672))
REPRESENTATION_CONTEXT('','3D')
);
#36668=(
GEOMETRIC_REPRESENTATION_CONTEXT(3)
GLOBAL_UNCERTAINTY_ASSIGNED_CONTEXT((#36656))
GLOBAL_UNIT_ASSIGNED_CONTEXT((#36669,#36671,#36672))
REPRESENTATION_CONTEXT('','3D')
);
#36669=(
LENGTH_UNIT()
NAMED_UNIT(*)
SI_UNIT(.MILLI.,.METRE.)
);
#36671=(
NAMED_UNIT(*)
PLANE_ANGLE_UNIT()
SI_UNIT($,.RADIAN.)
);
#36672=(
NAMED_UNIT(*)
SI_UNIT($,.STERADIAN.)
SOLID_ANGLE_UNIT()
);
#36677=SHAPE_DEFINITION_REPRESENTATION(#36688,#36709);
#36688=PRODUCT_DEFINITION_SHAPE('',$,#36721);
#36709=SHAPE_REPRESENTATION('',(#18564),#36661);
#36716=PRODUCT_DEFINITION_CONTEXT('part definition',#36751,'design');
#36721=PRODUCT_DEFINITION('Feed Head Aluminum Chassis',
'Feed Head Aluminum Chassis',#36732,#36716);
#36732=PRODUCT_DEFINITION_FORMATION('',$,#36757);
#36751=APPLICATION_CONTEXT(
'Core Data for Automotive Mechanical Design Process');
#36752=PRODUCT_CONTEXT('part definition',#36751,'mechanical');
#36757=PRODUCT('Feed Head Aluminum Chassis',
'Feed Head Aluminum Chassis',$,(#36752));
#36768=PRESENTATION_STYLE_ASSIGNMENT((#36775));
#36775=SURFACE_STYLE_USAGE(.BOTH.,#36782);
#36782=SURFACE_SIDE_STYLE('',(#36789));
#36789=SURFACE_STYLE_FILL_AREA(#36796);
#36796=FILL_AREA_STYLE('Opaque(21,23,26)',(#36803));
#36803=FILL_AREA_STYLE_COLOUR('Opaque(21,23,26)',#36810);
#36810=COLOUR_RGB('Opaque(21,23,26)',0.0823529411764706,0.0901960784313725,
0.101960784313725);
ENDSEC;
END-ISO-10303-21;
